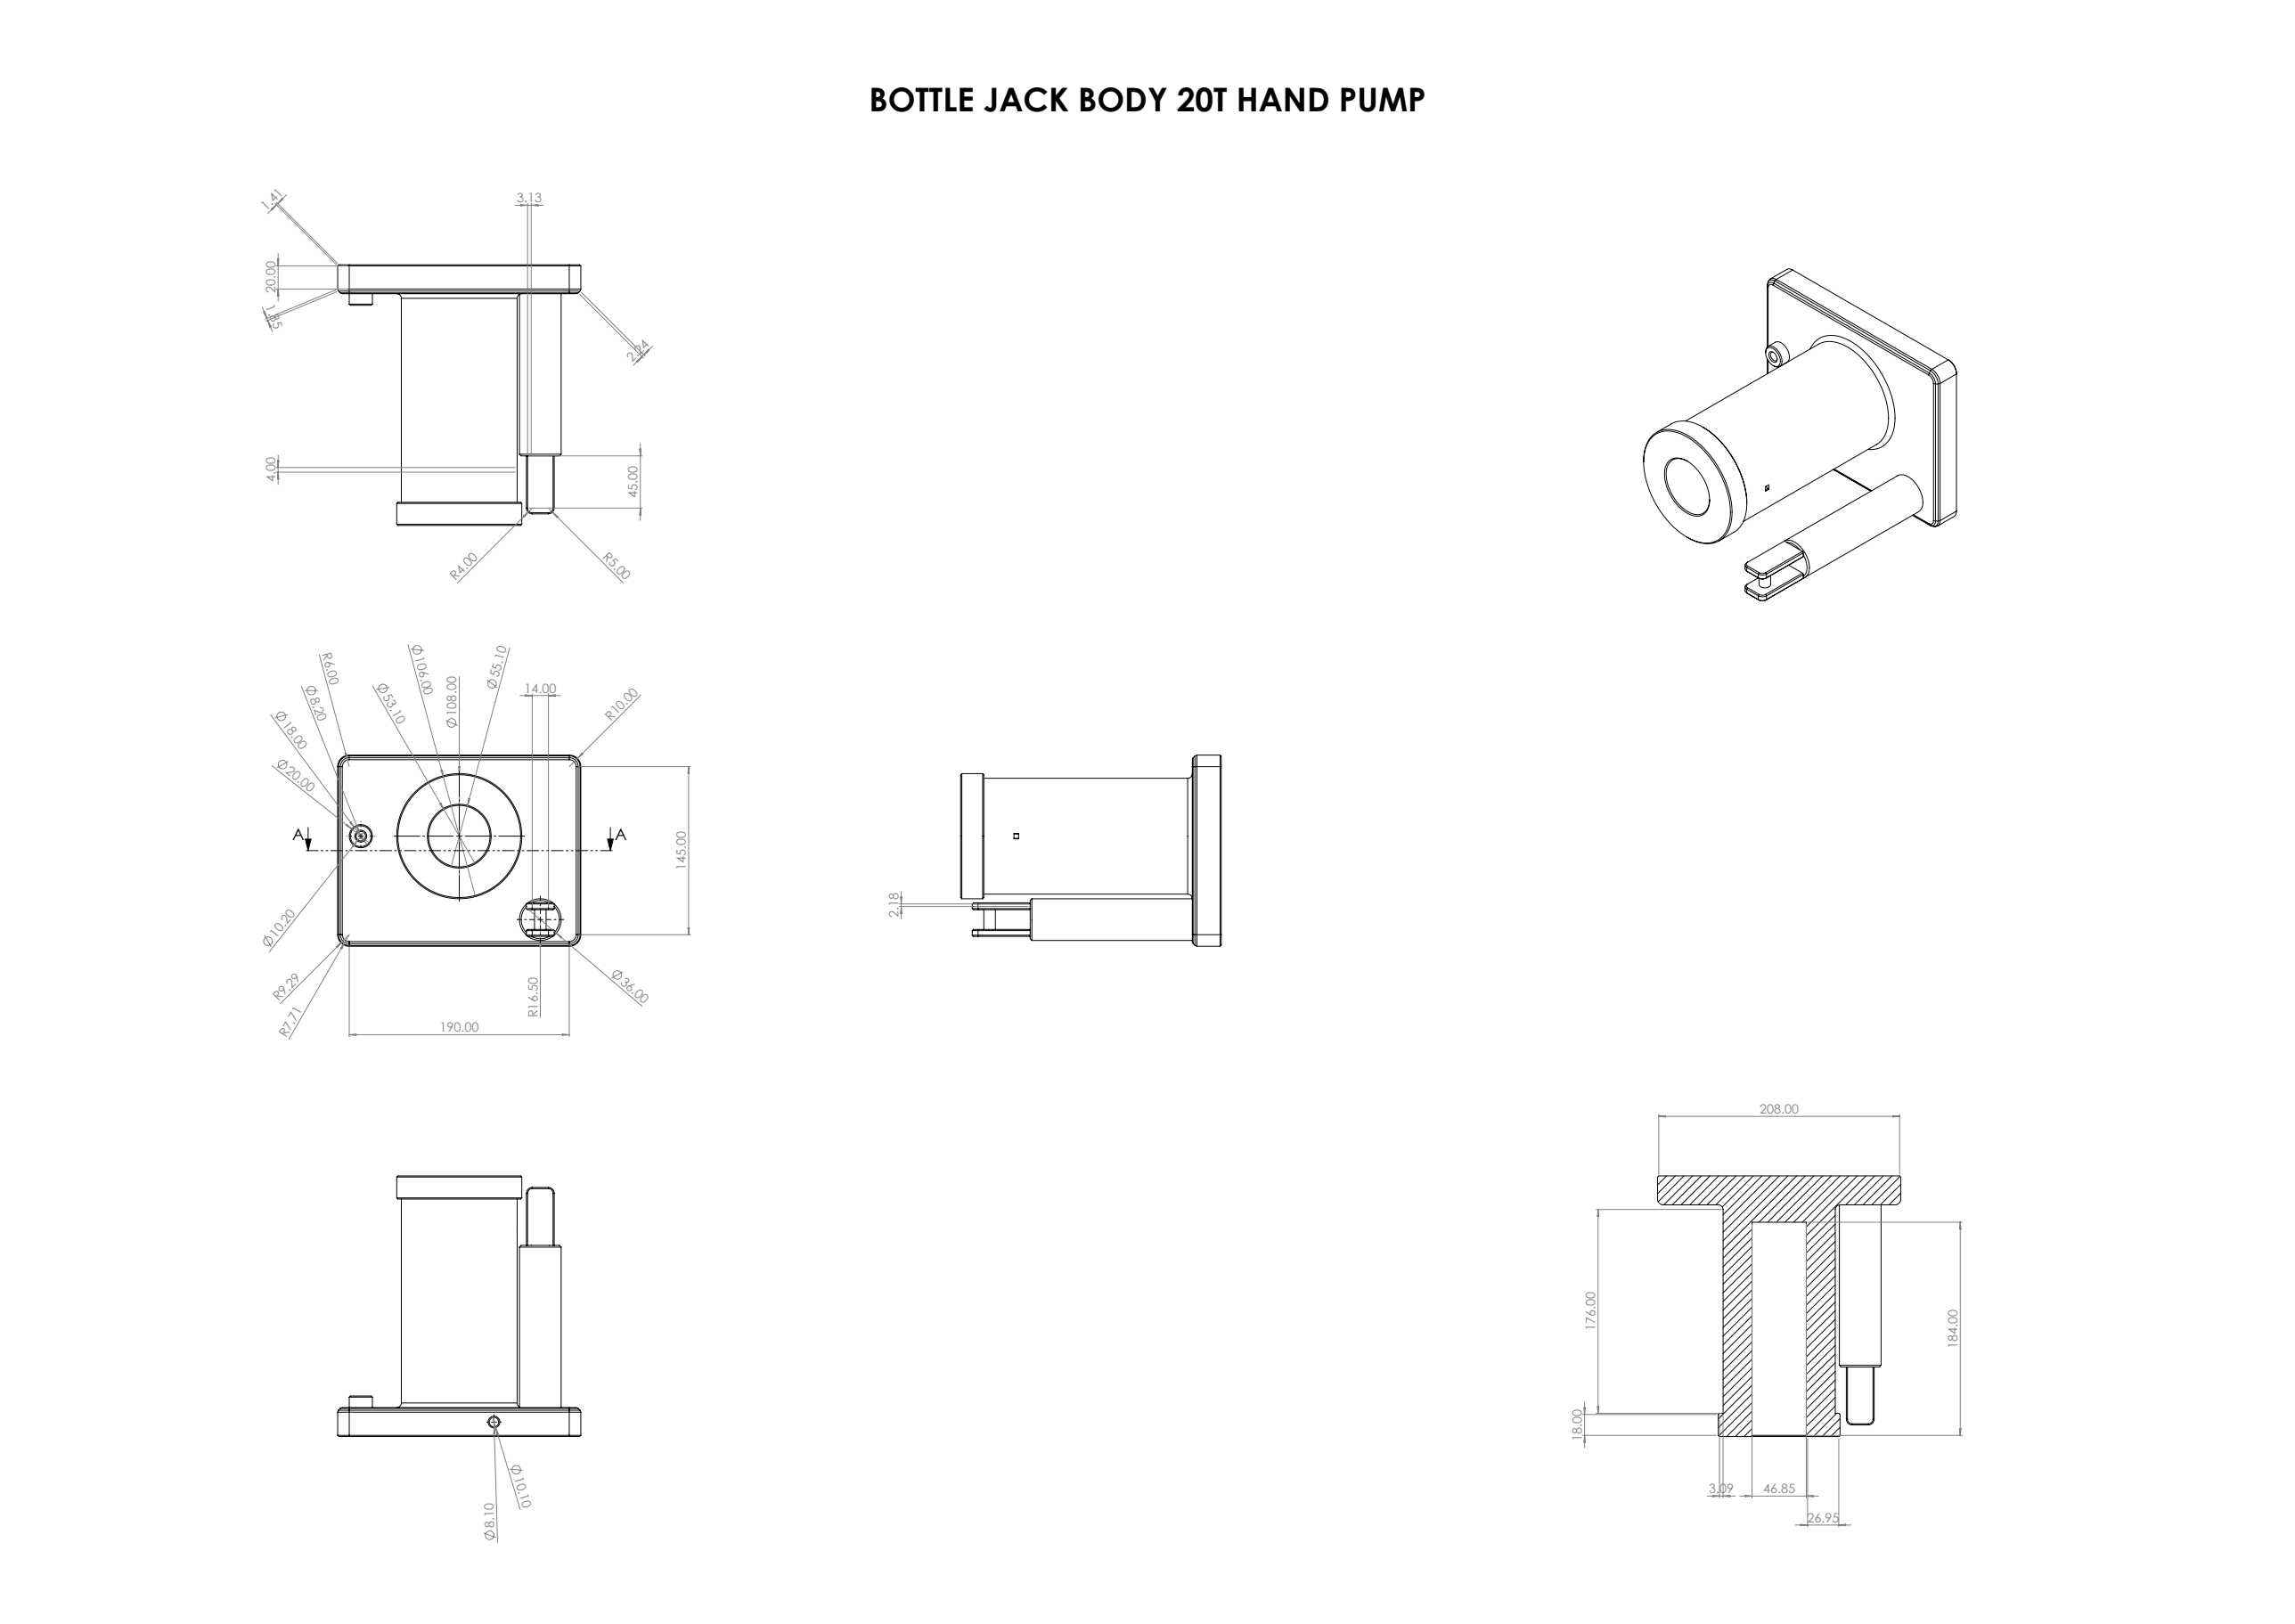
ISO-10303-21;
HEADER;
/* Generated by software containing ST-Developer
 * from STEP Tools, Inc. (www.steptools.com) 
 */

FILE_DESCRIPTION(
/* description */ (''),
/* implementation_level */ '2;1');

FILE_NAME(
/* name */ '09_Bottle_Jack_Body_20T_Hand_Pump.step',
/* time_stamp */ '2026-10-20T10:03:03-07:00',
/* author */ (''),
/* organization */ (''),
/* preprocessor_version */ 'ST-DEVELOPER v20.2',
/* originating_system */ 'Autodesk Translation Framework v15.15.0.0',
/* authorisation */ '');

FILE_SCHEMA (('AUTOMOTIVE_DESIGN { 1 0 10303 214 3 1 1 }'));
ENDSEC;

DATA;
#10=MECHANICAL_DESIGN_GEOMETRIC_PRESENTATION_REPRESENTATION('',(#528),#71492);
#376=TOROIDAL_SURFACE('',#29501,5.4,0.4);
#386=SHAPE_REPRESENTATION_RELATIONSHIP('SRR','None',#71607,#405);
#405=ADVANCED_BREP_SHAPE_REPRESENTATION('',(#424),#71477);
#424=MANIFOLD_SOLID_BREP('Jack body',#28463);
#528=STYLED_ITEM('',(#71866),#424);
#1575=CYLINDRICAL_SURFACE('',#29374,0.2);
#1576=CYLINDRICAL_SURFACE('',#29392,1.);
#1577=CYLINDRICAL_SURFACE('',#29395,1.);
#1578=CYLINDRICAL_SURFACE('',#29445,0.5);
#1579=CYLINDRICAL_SURFACE('',#29447,0.5);
#1580=CYLINDRICAL_SURFACE('',#29456,1.);
#1581=CYLINDRICAL_SURFACE('',#29459,0.41);
#1582=CYLINDRICAL_SURFACE('',#29463,0.405000000000001);
#1583=CYLINDRICAL_SURFACE('',#29467,0.5);
#1584=CYLINDRICAL_SURFACE('',#29468,0.5);
#1585=CYLINDRICAL_SURFACE('',#29470,0.5);
#1586=CYLINDRICAL_SURFACE('',#29488,1.8);
#1587=CYLINDRICAL_SURFACE('',#29492,2.655);
#1588=CYLINDRICAL_SURFACE('',#29505,5.);
#1589=CYLINDRICAL_SURFACE('',#29511,5.4);
#1590=CYLINDRICAL_SURFACE('',#29528,1.);
#1591=CYLINDRICAL_SURFACE('',#29533,1.);
#1918=FACE_BOUND('',#5174,.T.);
#1919=FACE_BOUND('',#5175,.T.);
#1920=FACE_BOUND('',#5176,.T.);
#1921=FACE_BOUND('',#5192,.T.);
#1922=FACE_BOUND('',#5208,.T.);
#1923=FACE_BOUND('',#5215,.T.);
#1924=FACE_BOUND('',#5229,.T.);
#1925=FACE_BOUND('',#5254,.T.);
#1926=FACE_BOUND('',#5260,.T.);
#1927=FACE_BOUND('',#5262,.T.);
#2238=CIRCLE('',#29348,0.770710678118652);
#2239=CIRCLE('',#29349,0.599999999999999);
#2240=CIRCLE('',#29352,0.770710678118652);
#2241=CIRCLE('',#29353,0.599999999999999);
#2242=CIRCLE('',#29356,0.770710678118652);
#2243=CIRCLE('',#29357,0.599999999999999);
#2244=CIRCLE('',#29360,0.770710678118652);
#2245=CIRCLE('',#29361,0.599999999999999);
#2246=CIRCLE('',#29365,0.929289321881342);
#2247=CIRCLE('',#29368,0.929289321881342);
#2248=CIRCLE('',#29370,5.4);
#2249=CIRCLE('',#29371,1.8);
#2250=CIRCLE('',#29372,1.);
#2251=CIRCLE('',#29375,0.2);
#2252=CIRCLE('',#29376,0.2);
#2253=CIRCLE('',#29380,1.);
#2254=CIRCLE('',#29383,0.929289321881336);
#2255=CIRCLE('',#29384,1.);
#2256=CIRCLE('',#29387,0.929289321881336);
#2257=CIRCLE('',#29388,1.);
#2258=CIRCLE('',#29391,1.);
#2259=CIRCLE('',#29393,1.);
#2260=CIRCLE('',#29396,1.);
#2261=CIRCLE('',#29398,0.504999999999995);
#2262=CIRCLE('',#29403,0.5);
#2263=CIRCLE('',#29404,0.400000000000011);
#2264=CIRCLE('',#29407,0.5);
#2265=CIRCLE('',#29408,0.400000000000012);
#2266=CIRCLE('',#29411,1.65);
#2267=CIRCLE('',#29415,0.5);
#2268=CIRCLE('',#29416,0.400000000000012);
#2269=CIRCLE('',#29419,0.5);
#2270=CIRCLE('',#29420,0.400000000000011);
#2271=CIRCLE('',#29423,0.5);
#2272=CIRCLE('',#29426,0.5);
#2273=CIRCLE('',#29427,0.400000000000011);
#2274=CIRCLE('',#29430,0.5);
#2275=CIRCLE('',#29431,0.400000000000012);
#2276=CIRCLE('',#29434,0.5);
#2277=CIRCLE('',#29437,0.5);
#2278=CIRCLE('',#29438,0.400000000000012);
#2279=CIRCLE('',#29441,0.5);
#2280=CIRCLE('',#29442,0.400000000000011);
#2281=CIRCLE('',#29450,1.65);
#2282=CIRCLE('',#29452,0.9);
#2283=CIRCLE('',#29453,1.);
#2284=CIRCLE('',#29455,0.51);
#2285=CIRCLE('',#29458,0.41);
#2286=CIRCLE('',#29460,0.41);
#2287=CIRCLE('',#29462,0.405000000000001);
#2288=CIRCLE('',#29464,0.405000000000001);
#2289=CIRCLE('',#29472,1.65);
#2290=CIRCLE('',#29476,1.65);
#2291=CIRCLE('',#29478,1.65);
#2292=CIRCLE('',#29481,1.65);
#2293=CIRCLE('',#29483,1.65);
#2294=CIRCLE('',#29484,1.65);
#2295=CIRCLE('',#29485,1.65);
#2296=CIRCLE('',#29487,1.8);
#2297=CIRCLE('',#29490,2.755);
#2298=CIRCLE('',#29491,2.655);
#2299=CIRCLE('',#29493,2.655);
#2300=CIRCLE('',#29495,5.3);
#2301=CIRCLE('',#29497,5.);
#2302=CIRCLE('',#29499,5.);
#2303=CIRCLE('',#29502,5.);
#2304=CIRCLE('',#29503,0.4);
#2305=CIRCLE('',#29504,5.);
#2306=CIRCLE('',#29506,5.);
#2307=CIRCLE('',#29508,5.3);
#2308=CIRCLE('',#29510,5.4);
#2309=CIRCLE('',#29512,5.4);
#2310=CIRCLE('',#29516,0.9);
#2311=CIRCLE('',#29519,1.);
#2312=CIRCLE('',#29520,0.9);
#2313=CIRCLE('',#29523,1.);
#2314=CIRCLE('',#29524,0.9);
#2315=CIRCLE('',#29527,0.9);
#2819=CONICAL_SURFACE('',#29347,0.685355339059325,1.17809724509615);
#2820=CONICAL_SURFACE('',#29351,0.685355339059325,1.17809724509615);
#2821=CONICAL_SURFACE('',#29355,0.685355339059325,1.17809724509615);
#2822=CONICAL_SURFACE('',#29359,0.685355339059325,1.17809724509615);
#2823=CONICAL_SURFACE('',#29364,0.85,0.785398163397452);
#2824=CONICAL_SURFACE('',#29367,0.85,0.785398163397452);
#2825=CONICAL_SURFACE('',#29379,0.964644660940671,0.392699081698743);
#2826=CONICAL_SURFACE('',#29382,0.964644660940668,0.392699081698775);
#2827=CONICAL_SURFACE('',#29386,0.964644660940668,0.392699081698775);
#2828=CONICAL_SURFACE('',#29390,0.964644660940671,0.392699081698743);
#2829=CONICAL_SURFACE('',#29399,0.85,0.785398163397452);
#2830=CONICAL_SURFACE('',#29402,0.450000000000006,0.785398163397392);
#2831=CONICAL_SURFACE('',#29406,0.450000000000006,0.785398163397389);
#2832=CONICAL_SURFACE('',#29414,0.450000000000006,0.785398163397389);
#2833=CONICAL_SURFACE('',#29418,0.450000000000006,0.785398163397392);
#2834=CONICAL_SURFACE('',#29425,0.450000000000006,0.785398163397392);
#2835=CONICAL_SURFACE('',#29429,0.450000000000006,0.785398163397389);
#2836=CONICAL_SURFACE('',#29436,0.450000000000006,0.785398163397389);
#2837=CONICAL_SURFACE('',#29440,0.450000000000006,0.785398163397392);
#2838=CONICAL_SURFACE('',#29451,0.95,0.785398163397475);
#2839=CONICAL_SURFACE('',#29457,0.46,0.785398163397475);
#2840=CONICAL_SURFACE('',#29461,0.454999999999998,0.785398163397422);
#2841=CONICAL_SURFACE('',#29465,0.405000000000001,1.02974425867666);
#2842=CONICAL_SURFACE('',#29466,0.205,1.02974425867666);
#2843=CONICAL_SURFACE('',#29486,1.725,0.785398163397431);
#2844=CONICAL_SURFACE('',#29489,2.705,0.785398163397477);
#2845=CONICAL_SURFACE('',#29509,5.35,0.785398163397479);
#2846=CONICAL_SURFACE('',#29513,5.35,0.785398163397479);
#2847=CONICAL_SURFACE('',#29515,0.95,0.785398163397475);
#2848=CONICAL_SURFACE('',#29518,0.95,0.785398163397475);
#2849=CONICAL_SURFACE('',#29522,0.95,0.785398163397475);
#2850=CONICAL_SURFACE('',#29526,0.95,0.785398163397475);
#2851=CONICAL_SURFACE('',#29531,0.85,0.785398163397452);
#3537=FACE_OUTER_BOUND('',#5161,.T.);
#3538=FACE_OUTER_BOUND('',#5162,.T.);
#3539=FACE_OUTER_BOUND('',#5163,.T.);
#3540=FACE_OUTER_BOUND('',#5164,.T.);
#3541=FACE_OUTER_BOUND('',#5165,.T.);
#3542=FACE_OUTER_BOUND('',#5166,.T.);
#3543=FACE_OUTER_BOUND('',#5167,.T.);
#3544=FACE_OUTER_BOUND('',#5168,.T.);
#3545=FACE_OUTER_BOUND('',#5169,.T.);
#3546=FACE_OUTER_BOUND('',#5170,.T.);
#3547=FACE_OUTER_BOUND('',#5171,.T.);
#3548=FACE_OUTER_BOUND('',#5172,.T.);
#3549=FACE_OUTER_BOUND('',#5173,.T.);
#3550=FACE_OUTER_BOUND('',#5177,.T.);
#3551=FACE_OUTER_BOUND('',#5178,.T.);
#3552=FACE_OUTER_BOUND('',#5179,.T.);
#3553=FACE_OUTER_BOUND('',#5180,.T.);
#3554=FACE_OUTER_BOUND('',#5181,.T.);
#3555=FACE_OUTER_BOUND('',#5182,.T.);
#3556=FACE_OUTER_BOUND('',#5183,.T.);
#3557=FACE_OUTER_BOUND('',#5184,.T.);
#3558=FACE_OUTER_BOUND('',#5185,.T.);
#3559=FACE_OUTER_BOUND('',#5186,.T.);
#3560=FACE_OUTER_BOUND('',#5187,.T.);
#3561=FACE_OUTER_BOUND('',#5188,.T.);
#3562=FACE_OUTER_BOUND('',#5189,.T.);
#3563=FACE_OUTER_BOUND('',#5190,.T.);
#3564=FACE_OUTER_BOUND('',#5191,.T.);
#3565=FACE_OUTER_BOUND('',#5193,.T.);
#3566=FACE_OUTER_BOUND('',#5194,.T.);
#3567=FACE_OUTER_BOUND('',#5195,.T.);
#3568=FACE_OUTER_BOUND('',#5196,.T.);
#3569=FACE_OUTER_BOUND('',#5197,.T.);
#3570=FACE_OUTER_BOUND('',#5198,.T.);
#3571=FACE_OUTER_BOUND('',#5199,.T.);
#3572=FACE_OUTER_BOUND('',#5200,.T.);
#3573=FACE_OUTER_BOUND('',#5201,.T.);
#3574=FACE_OUTER_BOUND('',#5202,.T.);
#3575=FACE_OUTER_BOUND('',#5203,.T.);
#3576=FACE_OUTER_BOUND('',#5204,.T.);
#3577=FACE_OUTER_BOUND('',#5205,.T.);
#3578=FACE_OUTER_BOUND('',#5206,.T.);
#3579=FACE_OUTER_BOUND('',#5207,.T.);
#3580=FACE_OUTER_BOUND('',#5209,.T.);
#3581=FACE_OUTER_BOUND('',#5210,.T.);
#3582=FACE_OUTER_BOUND('',#5211,.T.);
#3583=FACE_OUTER_BOUND('',#5212,.T.);
#3584=FACE_OUTER_BOUND('',#5213,.T.);
#3585=FACE_OUTER_BOUND('',#5214,.T.);
#3586=FACE_OUTER_BOUND('',#5216,.T.);
#3587=FACE_OUTER_BOUND('',#5217,.T.);
#3588=FACE_OUTER_BOUND('',#5218,.T.);
#3589=FACE_OUTER_BOUND('',#5219,.T.);
#3590=FACE_OUTER_BOUND('',#5220,.T.);
#3591=FACE_OUTER_BOUND('',#5221,.T.);
#3592=FACE_OUTER_BOUND('',#5222,.T.);
#3593=FACE_OUTER_BOUND('',#5223,.T.);
#3594=FACE_OUTER_BOUND('',#5224,.T.);
#3595=FACE_OUTER_BOUND('',#5225,.T.);
#3596=FACE_OUTER_BOUND('',#5226,.T.);
#3597=FACE_OUTER_BOUND('',#5227,.T.);
#3598=FACE_OUTER_BOUND('',#5228,.T.);
#3599=FACE_OUTER_BOUND('',#5230,.T.);
#3600=FACE_OUTER_BOUND('',#5231,.T.);
#3601=FACE_OUTER_BOUND('',#5232,.T.);
#3602=FACE_OUTER_BOUND('',#5233,.T.);
#3603=FACE_OUTER_BOUND('',#5234,.T.);
#3604=FACE_OUTER_BOUND('',#5235,.T.);
#3605=FACE_OUTER_BOUND('',#5236,.T.);
#3606=FACE_OUTER_BOUND('',#5237,.T.);
#3607=FACE_OUTER_BOUND('',#5238,.T.);
#3608=FACE_OUTER_BOUND('',#5239,.T.);
#3609=FACE_OUTER_BOUND('',#5240,.T.);
#3610=FACE_OUTER_BOUND('',#5241,.T.);
#3611=FACE_OUTER_BOUND('',#5242,.T.);
#3612=FACE_OUTER_BOUND('',#5243,.T.);
#3613=FACE_OUTER_BOUND('',#5244,.T.);
#3614=FACE_OUTER_BOUND('',#5245,.T.);
#3615=FACE_OUTER_BOUND('',#5246,.T.);
#3616=FACE_OUTER_BOUND('',#5247,.T.);
#3617=FACE_OUTER_BOUND('',#5248,.T.);
#3618=FACE_OUTER_BOUND('',#5249,.T.);
#3619=FACE_OUTER_BOUND('',#5250,.T.);
#3620=FACE_OUTER_BOUND('',#5251,.T.);
#3621=FACE_OUTER_BOUND('',#5252,.T.);
#3622=FACE_OUTER_BOUND('',#5253,.T.);
#3623=FACE_OUTER_BOUND('',#5255,.T.);
#3624=FACE_OUTER_BOUND('',#5256,.T.);
#3625=FACE_OUTER_BOUND('',#5257,.T.);
#3626=FACE_OUTER_BOUND('',#5258,.T.);
#3627=FACE_OUTER_BOUND('',#5259,.T.);
#3628=FACE_OUTER_BOUND('',#5261,.T.);
#3629=FACE_OUTER_BOUND('',#5263,.T.);
#3630=FACE_OUTER_BOUND('',#5264,.T.);
#3631=FACE_OUTER_BOUND('',#5265,.T.);
#3632=FACE_OUTER_BOUND('',#5266,.T.);
#3633=FACE_OUTER_BOUND('',#5267,.T.);
#3634=FACE_OUTER_BOUND('',#5268,.T.);
#3635=FACE_OUTER_BOUND('',#5269,.T.);
#3636=FACE_OUTER_BOUND('',#5270,.T.);
#3637=FACE_OUTER_BOUND('',#5271,.T.);
#3638=FACE_OUTER_BOUND('',#5272,.T.);
#3639=FACE_OUTER_BOUND('',#5273,.T.);
#3640=FACE_OUTER_BOUND('',#5274,.T.);
#3641=FACE_OUTER_BOUND('',#5275,.T.);
#3642=FACE_OUTER_BOUND('',#5276,.T.);
#3643=FACE_OUTER_BOUND('',#5277,.T.);
#3644=FACE_OUTER_BOUND('',#5278,.T.);
#3645=FACE_OUTER_BOUND('',#5279,.T.);
#3646=FACE_OUTER_BOUND('',#5280,.T.);
#5161=EDGE_LOOP('',(#20973,#20974,#20975,#20976));
#5162=EDGE_LOOP('',(#20977,#20978,#20979,#20980));
#5163=EDGE_LOOP('',(#20981,#20982,#20983,#20984));
#5164=EDGE_LOOP('',(#20985,#20986,#20987,#20988));
#5165=EDGE_LOOP('',(#20989,#20990,#20991,#20992));
#5166=EDGE_LOOP('',(#20993,#20994,#20995,#20996));
#5167=EDGE_LOOP('',(#20997,#20998,#20999,#21000));
#5168=EDGE_LOOP('',(#21001,#21002,#21003,#21004));
#5169=EDGE_LOOP('',(#21005,#21006,#21007,#21008));
#5170=EDGE_LOOP('',(#21009,#21010,#21011,#21012));
#5171=EDGE_LOOP('',(#21013,#21014,#21015,#21016));
#5172=EDGE_LOOP('',(#21017,#21018,#21019,#21020));
#5173=EDGE_LOOP('',(#21021,#21022,#21023,#21024,#21025,#21026,#21027,#21028));
#5174=EDGE_LOOP('',(#21029));
#5175=EDGE_LOOP('',(#21030));
#5176=EDGE_LOOP('',(#21031));
#5177=EDGE_LOOP('',(#21032,#21033,#21034,#21035));
#5178=EDGE_LOOP('',(#21036,#21037,#21038,#21039));
#5179=EDGE_LOOP('',(#21040,#21041,#21042,#21043));
#5180=EDGE_LOOP('',(#21044,#21045,#21046,#21047));
#5181=EDGE_LOOP('',(#21048,#21049,#21050,#21051));
#5182=EDGE_LOOP('',(#21052,#21053,#21054,#21055));
#5183=EDGE_LOOP('',(#21056,#21057,#21058,#21059));
#5184=EDGE_LOOP('',(#21060,#21061,#21062,#21063));
#5185=EDGE_LOOP('',(#21064,#21065,#21066,#21067));
#5186=EDGE_LOOP('',(#21068,#21069,#21070,#21071));
#5187=EDGE_LOOP('',(#21072,#21073,#21074,#21075));
#5188=EDGE_LOOP('',(#21076,#21077,#21078,#21079));
#5189=EDGE_LOOP('',(#21080,#21081,#21082,#21083));
#5190=EDGE_LOOP('',(#21084,#21085,#21086,#21087));
#5191=EDGE_LOOP('',(#21088,#21089,#21090,#21091));
#5192=EDGE_LOOP('',(#21092));
#5193=EDGE_LOOP('',(#21093,#21094,#21095,#21096));
#5194=EDGE_LOOP('',(#21097,#21098,#21099,#21100));
#5195=EDGE_LOOP('',(#21101,#21102,#21103,#21104));
#5196=EDGE_LOOP('',(#21105,#21106,#21107,#21108));
#5197=EDGE_LOOP('',(#21109,#21110,#21111,#21112));
#5198=EDGE_LOOP('',(#21113,#21114,#21115,#21116));
#5199=EDGE_LOOP('',(#21117,#21118,#21119,#21120));
#5200=EDGE_LOOP('',(#21121,#21122,#21123,#21124));
#5201=EDGE_LOOP('',(#21125,#21126,#21127,#21128,#21129,#21130,#21131,#21132));
#5202=EDGE_LOOP('',(#21133,#21134,#21135,#21136));
#5203=EDGE_LOOP('',(#21137,#21138,#21139,#21140));
#5204=EDGE_LOOP('',(#21141,#21142,#21143,#21144));
#5205=EDGE_LOOP('',(#21145,#21146,#21147,#21148));
#5206=EDGE_LOOP('',(#21149,#21150,#21151,#21152));
#5207=EDGE_LOOP('',(#21153,#21154,#21155,#21156,#21157,#21158));
#5208=EDGE_LOOP('',(#21159));
#5209=EDGE_LOOP('',(#21160,#21161,#21162,#21163));
#5210=EDGE_LOOP('',(#21164,#21165,#21166,#21167));
#5211=EDGE_LOOP('',(#21168,#21169,#21170,#21171));
#5212=EDGE_LOOP('',(#21172,#21173,#21174,#21175));
#5213=EDGE_LOOP('',(#21176,#21177,#21178,#21179));
#5214=EDGE_LOOP('',(#21180,#21181,#21182,#21183,#21184,#21185));
#5215=EDGE_LOOP('',(#21186));
#5216=EDGE_LOOP('',(#21187,#21188,#21189,#21190));
#5217=EDGE_LOOP('',(#21191,#21192,#21193,#21194));
#5218=EDGE_LOOP('',(#21195,#21196,#21197,#21198));
#5219=EDGE_LOOP('',(#21199,#21200,#21201,#21202));
#5220=EDGE_LOOP('',(#21203,#21204,#21205,#21206));
#5221=EDGE_LOOP('',(#21207,#21208,#21209,#21210,#21211));
#5222=EDGE_LOOP('',(#21212,#21213,#21214,#21215));
#5223=EDGE_LOOP('',(#21216,#21217,#21218,#21219));
#5224=EDGE_LOOP('',(#21220,#21221,#21222,#21223));
#5225=EDGE_LOOP('',(#21224,#21225,#21226,#21227,#21228));
#5226=EDGE_LOOP('',(#21229,#21230,#21231,#21232));
#5227=EDGE_LOOP('',(#21233,#21234,#21235,#21236));
#5228=EDGE_LOOP('',(#21237));
#5229=EDGE_LOOP('',(#21238));
#5230=EDGE_LOOP('',(#21239,#21240,#21241,#21242));
#5231=EDGE_LOOP('',(#21243,#21244,#21245,#21246));
#5232=EDGE_LOOP('',(#21247,#21248,#21249,#21250));
#5233=EDGE_LOOP('',(#21251,#21252,#21253,#21254));
#5234=EDGE_LOOP('',(#21255,#21256,#21257,#21258));
#5235=EDGE_LOOP('',(#21259,#21260,#21261));
#5236=EDGE_LOOP('',(#21262,#21263,#21264));
#5237=EDGE_LOOP('',(#21265,#21266,#21267,#21268));
#5238=EDGE_LOOP('',(#21269,#21270,#21271,#21272));
#5239=EDGE_LOOP('',(#21273,#21274,#21275,#21276));
#5240=EDGE_LOOP('',(#21277,#21278,#21279,#21280));
#5241=EDGE_LOOP('',(#21281,#21282,#21283,#21284));
#5242=EDGE_LOOP('',(#21285,#21286,#21287,#21288,#21289));
#5243=EDGE_LOOP('',(#21290,#21291,#21292,#21293,#21294));
#5244=EDGE_LOOP('',(#21295,#21296));
#5245=EDGE_LOOP('',(#21297,#21298,#21299,#21300));
#5246=EDGE_LOOP('',(#21301,#21302,#21303,#21304,#21305,#21306,#21307,#21308));
#5247=EDGE_LOOP('',(#21309,#21310));
#5248=EDGE_LOOP('',(#21311,#21312,#21313,#21314,#21315,#21316,#21317,#21318,
#21319,#21320,#21321,#21322,#21323));
#5249=EDGE_LOOP('',(#21324,#21325,#21326,#21327,#21328,#21329,#21330,#21331,
#21332,#21333,#21334,#21335));
#5250=EDGE_LOOP('',(#21336,#21337,#21338,#21339));
#5251=EDGE_LOOP('',(#21340,#21341,#21342,#21343));
#5252=EDGE_LOOP('',(#21344,#21345,#21346,#21347));
#5253=EDGE_LOOP('',(#21348));
#5254=EDGE_LOOP('',(#21349));
#5255=EDGE_LOOP('',(#21350,#21351,#21352,#21353));
#5256=EDGE_LOOP('',(#21354,#21355,#21356,#21357));
#5257=EDGE_LOOP('',(#21358));
#5258=EDGE_LOOP('',(#21359,#21360,#21361,#21362,#21363));
#5259=EDGE_LOOP('',(#21364,#21365,#21366,#21367,#21368));
#5260=EDGE_LOOP('',(#21369,#21370,#21371,#21372));
#5261=EDGE_LOOP('',(#21373));
#5262=EDGE_LOOP('',(#21374));
#5263=EDGE_LOOP('',(#21375,#21376,#21377,#21378));
#5264=EDGE_LOOP('',(#21379,#21380,#21381,#21382));
#5265=EDGE_LOOP('',(#21383,#21384,#21385,#21386));
#5266=EDGE_LOOP('',(#21387,#21388,#21389,#21390));
#5267=EDGE_LOOP('',(#21391,#21392,#21393,#21394));
#5268=EDGE_LOOP('',(#21395,#21396,#21397,#21398));
#5269=EDGE_LOOP('',(#21399,#21400,#21401,#21402));
#5270=EDGE_LOOP('',(#21403,#21404,#21405,#21406));
#5271=EDGE_LOOP('',(#21407,#21408,#21409,#21410));
#5272=EDGE_LOOP('',(#21411,#21412,#21413,#21414));
#5273=EDGE_LOOP('',(#21415,#21416,#21417,#21418));
#5274=EDGE_LOOP('',(#21419,#21420,#21421,#21422));
#5275=EDGE_LOOP('',(#21423,#21424,#21425,#21426,#21427,#21428,#21429,#21430));
#5276=EDGE_LOOP('',(#21431,#21432,#21433,#21434));
#5277=EDGE_LOOP('',(#21435,#21436,#21437,#21438));
#5278=EDGE_LOOP('',(#21439,#21440,#21441,#21442));
#5279=EDGE_LOOP('',(#21443,#21444,#21445,#21446));
#5280=EDGE_LOOP('',(#21447,#21448,#21449,#21450));
#7402=LINE('',#43533,#9890);
#7403=LINE('',#43537,#9891);
#7404=LINE('',#43542,#9892);
#7405=LINE('',#43543,#9893);
#7406=LINE('',#43544,#9894);
#7407=LINE('',#43548,#9895);
#7408=LINE('',#43554,#9896);
#7409=LINE('',#43555,#9897);
#7410=LINE('',#43556,#9898);
#7411=LINE('',#43560,#9899);
#7412=LINE('',#43566,#9900);
#7413=LINE('',#43567,#9901);
#7414=LINE('',#43568,#9902);
#7415=LINE('',#43572,#9903);
#7416=LINE('',#43576,#9904);
#7417=LINE('',#43577,#9905);
#7418=LINE('',#43580,#9906);
#7419=LINE('',#43582,#9907);
#7420=LINE('',#43583,#9908);
#7421=LINE('',#43586,#9909);
#7422=LINE('',#43590,#9910);
#7423=LINE('',#43591,#9911);
#7424=LINE('',#43594,#9912);
#7425=LINE('',#43606,#9913);
#7426=LINE('',#43608,#9914);
#7427=LINE('',#43610,#9915);
#7428=LINE('',#43611,#9916);
#7429=LINE('',#43616,#9917);
#7430=LINE('',#43620,#9918);
#7431=LINE('',#43622,#9919);
#7432=LINE('',#43623,#9920);
#7433=LINE('',#43626,#9921);
#7434=LINE('',#43628,#9922);
#7435=LINE('',#43629,#9923);
#7436=LINE('',#43632,#9924);
#7437=LINE('',#43636,#9925);
#7438=LINE('',#43637,#9926);
#7439=LINE('',#43641,#9927);
#7440=LINE('',#43647,#9928);
#7441=LINE('',#43648,#9929);
#7442=LINE('',#43649,#9930);
#7443=LINE('',#43653,#9931);
#7444=LINE('',#43658,#9932);
#7445=LINE('',#43659,#9933);
#7446=LINE('',#43660,#9934);
#7447=LINE('',#43665,#9935);
#7448=LINE('',#43668,#9936);
#7449=LINE('',#43671,#9937);
#7450=LINE('',#43672,#9938);
#7451=LINE('',#43675,#9939);
#7452=LINE('',#43679,#9940);
#7453=LINE('',#43680,#9941);
#7454=LINE('',#43684,#9942);
#7455=LINE('',#43685,#9943);
#7456=LINE('',#43690,#9944);
#7457=LINE('',#43692,#9945);
#7458=LINE('',#43694,#9946);
#7459=LINE('',#43695,#9947);
#7460=LINE('',#43699,#9948);
#7461=LINE('',#43705,#9949);
#7462=LINE('',#43706,#9950);
#7463=LINE('',#43707,#9951);
#7464=LINE('',#43711,#9952);
#7465=LINE('',#43717,#9953);
#7466=LINE('',#43718,#9954);
#7467=LINE('',#43719,#9955);
#7468=LINE('',#43722,#9956);
#7469=LINE('',#43725,#9957);
#7470=LINE('',#43728,#9958);
#7471=LINE('',#43729,#9959);
#7472=LINE('',#43733,#9960);
#7473=LINE('',#43735,#9961);
#7474=LINE('',#43737,#9962);
#7475=LINE('',#43738,#9963);
#7476=LINE('',#43742,#9964);
#7477=LINE('',#43748,#9965);
#7478=LINE('',#43749,#9966);
#7479=LINE('',#43750,#9967);
#7480=LINE('',#43754,#9968);
#7481=LINE('',#43760,#9969);
#7482=LINE('',#43761,#9970);
#7483=LINE('',#43762,#9971);
#7484=LINE('',#43764,#9972);
#7485=LINE('',#43770,#9973);
#7486=LINE('',#43772,#9974);
#7487=LINE('',#43774,#9975);
#7488=LINE('',#43775,#9976);
#7489=LINE('',#43779,#9977);
#7490=LINE('',#43785,#9978);
#7491=LINE('',#43786,#9979);
#7492=LINE('',#43787,#9980);
#7493=LINE('',#43791,#9981);
#7494=LINE('',#43797,#9982);
#7495=LINE('',#43798,#9983);
#7496=LINE('',#43799,#9984);
#7497=LINE('',#43801,#9985);
#7498=LINE('',#43807,#9986);
#7499=LINE('',#43809,#9987);
#7500=LINE('',#43811,#9988);
#7501=LINE('',#43812,#9989);
#7502=LINE('',#43816,#9990);
#7503=LINE('',#43822,#9991);
#7504=LINE('',#43823,#9992);
#7505=LINE('',#43824,#9993);
#7506=LINE('',#43828,#9994);
#7507=LINE('',#43834,#9995);
#7508=LINE('',#43835,#9996);
#7509=LINE('',#43836,#9997);
#7510=LINE('',#43839,#9998);
#7511=LINE('',#43840,#9999);
#7512=LINE('',#43841,#10000);
#7513=LINE('',#43843,#10001);
#7514=LINE('',#43845,#10002);
#7515=LINE('',#43847,#10003);
#7516=LINE('',#43850,#10004);
#7517=LINE('',#43851,#10005);
#7518=LINE('',#43854,#10006);
#7519=LINE('',#43860,#10007);
#7520=LINE('',#43866,#10008);
#7521=LINE('',#43869,#10009);
#7522=LINE('',#43874,#10010);
#7523=LINE('',#43877,#10011);
#7524=LINE('',#43881,#10012);
#7525=LINE('',#43885,#10013);
#7526=LINE('',#43888,#10014);
#7527=LINE('',#43890,#10015);
#7528=LINE('',#43892,#10016);
#7529=LINE('',#43893,#10017);
#7530=LINE('',#43895,#10018);
#7531=LINE('',#43897,#10019);
#7532=LINE('',#43900,#10020);
#7533=LINE('',#43903,#10021);
#7534=LINE('',#43905,#10022);
#7535=LINE('',#43911,#10023);
#7536=LINE('',#43913,#10024);
#7537=LINE('',#43923,#10025);
#7538=LINE('',#43926,#10026);
#7539=LINE('',#43931,#10027);
#7540=LINE('',#43936,#10028);
#7541=LINE('',#43954,#10029);
#7542=LINE('',#43961,#10030);
#7543=LINE('',#43965,#10031);
#7544=LINE('',#43967,#10032);
#7545=LINE('',#43970,#10033);
#7546=LINE('',#43972,#10034);
#7547=LINE('',#43973,#10035);
#7548=LINE('',#43976,#10036);
#7549=LINE('',#43981,#10037);
#7550=LINE('',#43982,#10038);
#7551=LINE('',#43983,#10039);
#7552=LINE('',#43987,#10040);
#7553=LINE('',#43993,#10041);
#7554=LINE('',#43994,#10042);
#7555=LINE('',#43995,#10043);
#7556=LINE('',#43998,#10044);
#7557=LINE('',#44003,#10045);
#7558=LINE('',#44004,#10046);
#7559=LINE('',#44008,#10047);
#7560=LINE('',#44011,#10048);
#7561=LINE('',#44014,#10049);
#7562=LINE('',#44016,#10050);
#9890=VECTOR('',#33275,1.);
#9891=VECTOR('',#33278,1.);
#9892=VECTOR('',#33283,1.);
#9893=VECTOR('',#33284,1.);
#9894=VECTOR('',#33285,1.);
#9895=VECTOR('',#33288,1.);
#9896=VECTOR('',#33295,1.);
#9897=VECTOR('',#33296,1.);
#9898=VECTOR('',#33297,1.);
#9899=VECTOR('',#33300,1.);
#9900=VECTOR('',#33307,1.);
#9901=VECTOR('',#33308,1.);
#9902=VECTOR('',#33309,1.);
#9903=VECTOR('',#33312,1.);
#9904=VECTOR('',#33319,1.);
#9905=VECTOR('',#33320,1.);
#9906=VECTOR('',#33323,1.);
#9907=VECTOR('',#33324,1.);
#9908=VECTOR('',#33325,1.);
#9909=VECTOR('',#33328,1.);
#9910=VECTOR('',#33333,1.);
#9911=VECTOR('',#33334,1.);
#9912=VECTOR('',#33337,1.);
#9913=VECTOR('',#33350,1.);
#9914=VECTOR('',#33351,1.);
#9915=VECTOR('',#33352,1.);
#9916=VECTOR('',#33353,1.);
#9917=VECTOR('',#33358,1.);
#9918=VECTOR('',#33363,1.);
#9919=VECTOR('',#33364,1.);
#9920=VECTOR('',#33365,1.);
#9921=VECTOR('',#33368,1.);
#9922=VECTOR('',#33369,1.);
#9923=VECTOR('',#33370,1.);
#9924=VECTOR('',#33373,1.);
#9925=VECTOR('',#33378,1.);
#9926=VECTOR('',#33379,1.);
#9927=VECTOR('',#33382,1.);
#9928=VECTOR('',#33389,1.);
#9929=VECTOR('',#33390,1.);
#9930=VECTOR('',#33391,1.);
#9931=VECTOR('',#33394,1.);
#9932=VECTOR('',#33401,1.);
#9933=VECTOR('',#33402,1.);
#9934=VECTOR('',#33403,1.);
#9935=VECTOR('',#33410,1.);
#9936=VECTOR('',#33413,1.);
#9937=VECTOR('',#33416,1.);
#9938=VECTOR('',#33417,1.);
#9939=VECTOR('',#33420,1.);
#9940=VECTOR('',#33425,1.);
#9941=VECTOR('',#33426,1.);
#9942=VECTOR('',#33431,1.);
#9943=VECTOR('',#33432,1.);
#9944=VECTOR('',#33437,1.);
#9945=VECTOR('',#33438,1.);
#9946=VECTOR('',#33439,1.);
#9947=VECTOR('',#33440,1.);
#9948=VECTOR('',#33443,1.);
#9949=VECTOR('',#33450,1.);
#9950=VECTOR('',#33451,1.);
#9951=VECTOR('',#33452,1.);
#9952=VECTOR('',#33455,1.);
#9953=VECTOR('',#33462,1.);
#9954=VECTOR('',#33463,1.);
#9955=VECTOR('',#33464,1.);
#9956=VECTOR('',#33467,1.);
#9957=VECTOR('',#33470,1.);
#9958=VECTOR('',#33473,1.);
#9959=VECTOR('',#33474,1.);
#9960=VECTOR('',#33477,1.);
#9961=VECTOR('',#33478,1.);
#9962=VECTOR('',#33479,1.);
#9963=VECTOR('',#33480,1.);
#9964=VECTOR('',#33483,1.);
#9965=VECTOR('',#33490,1.);
#9966=VECTOR('',#33491,1.);
#9967=VECTOR('',#33492,1.);
#9968=VECTOR('',#33495,1.);
#9969=VECTOR('',#33502,1.);
#9970=VECTOR('',#33503,1.);
#9971=VECTOR('',#33504,1.);
#9972=VECTOR('',#33507,1.);
#9973=VECTOR('',#33512,1.);
#9974=VECTOR('',#33513,1.);
#9975=VECTOR('',#33514,1.);
#9976=VECTOR('',#33515,1.);
#9977=VECTOR('',#33518,1.);
#9978=VECTOR('',#33525,1.);
#9979=VECTOR('',#33526,1.);
#9980=VECTOR('',#33527,1.);
#9981=VECTOR('',#33530,1.);
#9982=VECTOR('',#33537,1.);
#9983=VECTOR('',#33538,1.);
#9984=VECTOR('',#33539,1.);
#9985=VECTOR('',#33542,1.);
#9986=VECTOR('',#33547,1.);
#9987=VECTOR('',#33548,1.);
#9988=VECTOR('',#33549,1.);
#9989=VECTOR('',#33550,1.);
#9990=VECTOR('',#33553,1.);
#9991=VECTOR('',#33560,1.);
#9992=VECTOR('',#33561,1.);
#9993=VECTOR('',#33562,1.);
#9994=VECTOR('',#33565,1.);
#9995=VECTOR('',#33572,1.);
#9996=VECTOR('',#33573,1.);
#9997=VECTOR('',#33574,1.);
#9998=VECTOR('',#33577,1.);
#9999=VECTOR('',#33578,1.);
#10000=VECTOR('',#33579,1.);
#10001=VECTOR('',#33582,1.);
#10002=VECTOR('',#33585,1.);
#10003=VECTOR('',#33588,1.);
#10004=VECTOR('',#33591,1.);
#10005=VECTOR('',#33592,1.);
#10006=VECTOR('',#33595,1.);
#10007=VECTOR('',#33602,0.95);
#10008=VECTOR('',#33611,1.);
#10009=VECTOR('',#33614,0.46);
#10010=VECTOR('',#33621,0.41);
#10011=VECTOR('',#33624,0.454999999999998);
#10012=VECTOR('',#33629,0.405000000000001);
#10013=VECTOR('',#33634,0.405000000000001);
#10014=VECTOR('',#33637,0.205);
#10015=VECTOR('',#33640,0.5);
#10016=VECTOR('',#33643,1.);
#10017=VECTOR('',#33644,1.);
#10018=VECTOR('',#33647,1.);
#10019=VECTOR('',#33650,1.);
#10020=VECTOR('',#33653,1.);
#10021=VECTOR('',#33658,1.);
#10022=VECTOR('',#33661,1.);
#10023=VECTOR('',#33670,1.);
#10024=VECTOR('',#33673,1.);
#10025=VECTOR('',#33688,1.725);
#10026=VECTOR('',#33693,1.8);
#10027=VECTOR('',#33698,2.705);
#10028=VECTOR('',#33705,2.655);
#10029=VECTOR('',#33732,5.);
#10030=VECTOR('',#33741,5.35);
#10031=VECTOR('',#33746,5.4);
#10032=VECTOR('',#33749,5.35);
#10033=VECTOR('',#33752,1.);
#10034=VECTOR('',#33753,1.);
#10035=VECTOR('',#33754,1.);
#10036=VECTOR('',#33757,1.);
#10037=VECTOR('',#33762,1.);
#10038=VECTOR('',#33763,1.);
#10039=VECTOR('',#33764,1.);
#10040=VECTOR('',#33767,1.);
#10041=VECTOR('',#33774,1.);
#10042=VECTOR('',#33775,1.);
#10043=VECTOR('',#33776,1.);
#10044=VECTOR('',#33779,1.);
#10045=VECTOR('',#33786,1.);
#10046=VECTOR('',#33787,1.);
#10047=VECTOR('',#33794,1.);
#10048=VECTOR('',#33799,1.);
#10049=VECTOR('',#33804,1.);
#10050=VECTOR('',#33807,1.);
#12235=VERTEX_POINT('',#43531);
#12236=VERTEX_POINT('',#43532);
#12237=VERTEX_POINT('',#43534);
#12238=VERTEX_POINT('',#43536);
#12239=VERTEX_POINT('',#43540);
#12240=VERTEX_POINT('',#43541);
#12241=VERTEX_POINT('',#43546);
#12242=VERTEX_POINT('',#43547);
#12243=VERTEX_POINT('',#43552);
#12244=VERTEX_POINT('',#43553);
#12245=VERTEX_POINT('',#43558);
#12246=VERTEX_POINT('',#43559);
#12247=VERTEX_POINT('',#43564);
#12248=VERTEX_POINT('',#43565);
#12249=VERTEX_POINT('',#43570);
#12250=VERTEX_POINT('',#43571);
#12251=VERTEX_POINT('',#43579);
#12252=VERTEX_POINT('',#43581);
#12253=VERTEX_POINT('',#43585);
#12254=VERTEX_POINT('',#43589);
#12255=VERTEX_POINT('',#43593);
#12256=VERTEX_POINT('',#43597);
#12257=VERTEX_POINT('',#43599);
#12258=VERTEX_POINT('',#43601);
#12259=VERTEX_POINT('',#43604);
#12260=VERTEX_POINT('',#43605);
#12261=VERTEX_POINT('',#43607);
#12262=VERTEX_POINT('',#43609);
#12263=VERTEX_POINT('',#43613);
#12264=VERTEX_POINT('',#43615);
#12265=VERTEX_POINT('',#43619);
#12266=VERTEX_POINT('',#43621);
#12267=VERTEX_POINT('',#43625);
#12268=VERTEX_POINT('',#43627);
#12269=VERTEX_POINT('',#43631);
#12270=VERTEX_POINT('',#43635);
#12271=VERTEX_POINT('',#43639);
#12272=VERTEX_POINT('',#43640);
#12273=VERTEX_POINT('',#43645);
#12274=VERTEX_POINT('',#43646);
#12275=VERTEX_POINT('',#43651);
#12276=VERTEX_POINT('',#43652);
#12277=VERTEX_POINT('',#43657);
#12278=VERTEX_POINT('',#43664);
#12279=VERTEX_POINT('',#43666);
#12280=VERTEX_POINT('',#43670);
#12281=VERTEX_POINT('',#43674);
#12282=VERTEX_POINT('',#43678);
#12283=VERTEX_POINT('',#43681);
#12284=VERTEX_POINT('',#43688);
#12285=VERTEX_POINT('',#43689);
#12286=VERTEX_POINT('',#43691);
#12287=VERTEX_POINT('',#43693);
#12288=VERTEX_POINT('',#43697);
#12289=VERTEX_POINT('',#43698);
#12290=VERTEX_POINT('',#43703);
#12291=VERTEX_POINT('',#43704);
#12292=VERTEX_POINT('',#43709);
#12293=VERTEX_POINT('',#43710);
#12294=VERTEX_POINT('',#43715);
#12295=VERTEX_POINT('',#43716);
#12296=VERTEX_POINT('',#43721);
#12297=VERTEX_POINT('',#43723);
#12298=VERTEX_POINT('',#43727);
#12299=VERTEX_POINT('',#43731);
#12300=VERTEX_POINT('',#43732);
#12301=VERTEX_POINT('',#43734);
#12302=VERTEX_POINT('',#43736);
#12303=VERTEX_POINT('',#43740);
#12304=VERTEX_POINT('',#43741);
#12305=VERTEX_POINT('',#43746);
#12306=VERTEX_POINT('',#43747);
#12307=VERTEX_POINT('',#43752);
#12308=VERTEX_POINT('',#43753);
#12309=VERTEX_POINT('',#43758);
#12310=VERTEX_POINT('',#43759);
#12311=VERTEX_POINT('',#43765);
#12312=VERTEX_POINT('',#43768);
#12313=VERTEX_POINT('',#43769);
#12314=VERTEX_POINT('',#43771);
#12315=VERTEX_POINT('',#43773);
#12316=VERTEX_POINT('',#43777);
#12317=VERTEX_POINT('',#43778);
#12318=VERTEX_POINT('',#43783);
#12319=VERTEX_POINT('',#43784);
#12320=VERTEX_POINT('',#43789);
#12321=VERTEX_POINT('',#43790);
#12322=VERTEX_POINT('',#43795);
#12323=VERTEX_POINT('',#43796);
#12324=VERTEX_POINT('',#43802);
#12325=VERTEX_POINT('',#43805);
#12326=VERTEX_POINT('',#43806);
#12327=VERTEX_POINT('',#43808);
#12328=VERTEX_POINT('',#43810);
#12329=VERTEX_POINT('',#43814);
#12330=VERTEX_POINT('',#43815);
#12331=VERTEX_POINT('',#43820);
#12332=VERTEX_POINT('',#43821);
#12333=VERTEX_POINT('',#43826);
#12334=VERTEX_POINT('',#43827);
#12335=VERTEX_POINT('',#43832);
#12336=VERTEX_POINT('',#43833);
#12337=VERTEX_POINT('',#43838);
#12338=VERTEX_POINT('',#43849);
#12339=VERTEX_POINT('',#43853);
#12340=VERTEX_POINT('',#43857);
#12341=VERTEX_POINT('',#43859);
#12342=VERTEX_POINT('',#43863);
#12343=VERTEX_POINT('',#43868);
#12344=VERTEX_POINT('',#43872);
#12345=VERTEX_POINT('',#43876);
#12346=VERTEX_POINT('',#43880);
#12347=VERTEX_POINT('',#43884);
#12348=VERTEX_POINT('',#43887);
#12349=VERTEX_POINT('',#43899);
#12350=VERTEX_POINT('',#43909);
#12351=VERTEX_POINT('',#43917);
#12352=VERTEX_POINT('',#43922);
#12353=VERTEX_POINT('',#43928);
#12354=VERTEX_POINT('',#43930);
#12355=VERTEX_POINT('',#43934);
#12356=VERTEX_POINT('',#43938);
#12357=VERTEX_POINT('',#43946);
#12358=VERTEX_POINT('',#43947);
#12359=VERTEX_POINT('',#43952);
#12360=VERTEX_POINT('',#43956);
#12361=VERTEX_POINT('',#43959);
#12362=VERTEX_POINT('',#43963);
#12363=VERTEX_POINT('',#43969);
#12364=VERTEX_POINT('',#43971);
#12365=VERTEX_POINT('',#43975);
#12366=VERTEX_POINT('',#43979);
#12367=VERTEX_POINT('',#43980);
#12368=VERTEX_POINT('',#43985);
#12369=VERTEX_POINT('',#43986);
#12370=VERTEX_POINT('',#43991);
#12371=VERTEX_POINT('',#43992);
#12372=VERTEX_POINT('',#43997);
#12373=VERTEX_POINT('',#44002);
#15370=EDGE_CURVE('',#12235,#12236,#7402,.T.);
#15371=EDGE_CURVE('',#12236,#12237,#2238,.T.);
#15372=EDGE_CURVE('',#12237,#12238,#7403,.T.);
#15373=EDGE_CURVE('',#12238,#12235,#2239,.T.);
#15374=EDGE_CURVE('',#12239,#12240,#7404,.T.);
#15375=EDGE_CURVE('',#12240,#12236,#7405,.T.);
#15376=EDGE_CURVE('',#12235,#12239,#7406,.T.);
#15377=EDGE_CURVE('',#12241,#12242,#7407,.T.);
#15378=EDGE_CURVE('',#12242,#12240,#2240,.T.);
#15379=EDGE_CURVE('',#12239,#12241,#2241,.T.);
#15380=EDGE_CURVE('',#12243,#12244,#7408,.T.);
#15381=EDGE_CURVE('',#12244,#12242,#7409,.T.);
#15382=EDGE_CURVE('',#12241,#12243,#7410,.T.);
#15383=EDGE_CURVE('',#12245,#12246,#7411,.T.);
#15384=EDGE_CURVE('',#12246,#12244,#2242,.T.);
#15385=EDGE_CURVE('',#12243,#12245,#2243,.T.);
#15386=EDGE_CURVE('',#12247,#12248,#7412,.T.);
#15387=EDGE_CURVE('',#12248,#12246,#7413,.T.);
#15388=EDGE_CURVE('',#12245,#12247,#7414,.T.);
#15389=EDGE_CURVE('',#12249,#12250,#7415,.T.);
#15390=EDGE_CURVE('',#12250,#12248,#2244,.T.);
#15391=EDGE_CURVE('',#12247,#12249,#2245,.T.);
#15392=EDGE_CURVE('',#12237,#12250,#7416,.T.);
#15393=EDGE_CURVE('',#12249,#12238,#7417,.T.);
#15394=EDGE_CURVE('',#12248,#12251,#7418,.T.);
#15395=EDGE_CURVE('',#12252,#12251,#7419,.T.);
#15396=EDGE_CURVE('',#12246,#12252,#7420,.T.);
#15397=EDGE_CURVE('',#12250,#12253,#7421,.T.);
#15398=EDGE_CURVE('',#12251,#12253,#2246,.T.);
#15399=EDGE_CURVE('',#12254,#12237,#7422,.T.);
#15400=EDGE_CURVE('',#12253,#12254,#7423,.T.);
#15401=EDGE_CURVE('',#12236,#12255,#7424,.T.);
#15402=EDGE_CURVE('',#12254,#12255,#2247,.T.);
#15403=EDGE_CURVE('',#12256,#12256,#2248,.T.);
#15404=EDGE_CURVE('',#12257,#12257,#2249,.T.);
#15405=EDGE_CURVE('',#12258,#12258,#2250,.T.);
#15406=EDGE_CURVE('',#12259,#12260,#7425,.F.);
#15407=EDGE_CURVE('',#12260,#12261,#7426,.T.);
#15408=EDGE_CURVE('',#12261,#12262,#7427,.F.);
#15409=EDGE_CURVE('',#12262,#12259,#7428,.T.);
#15410=EDGE_CURVE('',#12260,#12263,#2251,.T.);
#15411=EDGE_CURVE('',#12264,#12263,#7429,.T.);
#15412=EDGE_CURVE('',#12261,#12264,#2252,.T.);
#15413=EDGE_CURVE('',#12265,#12264,#7430,.F.);
#15414=EDGE_CURVE('',#12263,#12266,#7431,.F.);
#15415=EDGE_CURVE('',#12266,#12265,#7432,.T.);
#15416=EDGE_CURVE('',#12267,#12253,#7433,.T.);
#15417=EDGE_CURVE('',#12254,#12268,#7434,.T.);
#15418=EDGE_CURVE('',#12268,#12267,#7435,.T.);
#15419=EDGE_CURVE('',#12269,#12251,#7436,.T.);
#15420=EDGE_CURVE('',#12267,#12269,#2253,.T.);
#15421=EDGE_CURVE('',#12270,#12252,#7437,.T.);
#15422=EDGE_CURVE('',#12269,#12270,#7438,.T.);
#15423=EDGE_CURVE('',#12271,#12272,#7439,.T.);
#15424=EDGE_CURVE('',#12272,#12252,#2254,.T.);
#15425=EDGE_CURVE('',#12270,#12271,#2255,.T.);
#15426=EDGE_CURVE('',#12273,#12274,#7440,.T.);
#15427=EDGE_CURVE('',#12274,#12272,#7441,.T.);
#15428=EDGE_CURVE('',#12271,#12273,#7442,.T.);
#15429=EDGE_CURVE('',#12275,#12276,#7443,.T.);
#15430=EDGE_CURVE('',#12276,#12274,#2256,.T.);
#15431=EDGE_CURVE('',#12273,#12275,#2257,.T.);
#15432=EDGE_CURVE('',#12277,#12255,#7444,.T.);
#15433=EDGE_CURVE('',#12255,#12276,#7445,.T.);
#15434=EDGE_CURVE('',#12275,#12277,#7446,.T.);
#15435=EDGE_CURVE('',#12277,#12268,#2258,.T.);
#15436=EDGE_CURVE('',#12270,#12278,#7447,.T.);
#15437=EDGE_CURVE('',#12279,#12278,#2259,.T.);
#15438=EDGE_CURVE('',#12279,#12271,#7448,.T.);
#15439=EDGE_CURVE('',#12280,#12269,#7449,.T.);
#15440=EDGE_CURVE('',#12278,#12280,#7450,.T.);
#15441=EDGE_CURVE('',#12267,#12281,#7451,.T.);
#15442=EDGE_CURVE('',#12280,#12281,#2260,.T.);
#15443=EDGE_CURVE('',#12282,#12268,#7452,.T.);
#15444=EDGE_CURVE('',#12281,#12282,#7453,.T.);
#15445=EDGE_CURVE('',#12283,#12283,#2261,.T.);
#15446=EDGE_CURVE('',#12242,#12274,#7454,.T.);
#15447=EDGE_CURVE('',#12240,#12276,#7455,.T.);
#15448=EDGE_CURVE('',#12284,#12285,#7456,.T.);
#15449=EDGE_CURVE('',#12285,#12286,#7457,.T.);
#15450=EDGE_CURVE('',#12286,#12287,#7458,.T.);
#15451=EDGE_CURVE('',#12287,#12284,#7459,.T.);
#15452=EDGE_CURVE('',#12288,#12289,#7460,.T.);
#15453=EDGE_CURVE('',#12289,#12287,#2262,.T.);
#15454=EDGE_CURVE('',#12286,#12288,#2263,.T.);
#15455=EDGE_CURVE('',#12290,#12291,#7461,.T.);
#15456=EDGE_CURVE('',#12291,#12289,#7462,.T.);
#15457=EDGE_CURVE('',#12288,#12290,#7463,.T.);
#15458=EDGE_CURVE('',#12292,#12293,#7464,.T.);
#15459=EDGE_CURVE('',#12293,#12291,#2264,.T.);
#15460=EDGE_CURVE('',#12290,#12292,#2265,.T.);
#15461=EDGE_CURVE('',#12294,#12295,#7465,.T.);
#15462=EDGE_CURVE('',#12295,#12293,#7466,.T.);
#15463=EDGE_CURVE('',#12292,#12294,#7467,.T.);
#15464=EDGE_CURVE('',#12296,#12294,#7468,.T.);
#15465=EDGE_CURVE('',#12297,#12296,#2266,.T.);
#15466=EDGE_CURVE('',#12295,#12297,#7469,.T.);
#15467=EDGE_CURVE('',#12285,#12298,#7470,.T.);
#15468=EDGE_CURVE('',#12296,#12298,#7471,.T.);
#15469=EDGE_CURVE('',#12299,#12300,#7472,.F.);
#15470=EDGE_CURVE('',#12300,#12301,#7473,.T.);
#15471=EDGE_CURVE('',#12301,#12302,#7474,.T.);
#15472=EDGE_CURVE('',#12302,#12299,#7475,.T.);
#15473=EDGE_CURVE('',#12303,#12304,#7476,.T.);
#15474=EDGE_CURVE('',#12304,#12302,#2267,.T.);
#15475=EDGE_CURVE('',#12301,#12303,#2268,.T.);
#15476=EDGE_CURVE('',#12305,#12306,#7477,.T.);
#15477=EDGE_CURVE('',#12306,#12304,#7478,.T.);
#15478=EDGE_CURVE('',#12303,#12305,#7479,.T.);
#15479=EDGE_CURVE('',#12307,#12308,#7480,.T.);
#15480=EDGE_CURVE('',#12308,#12306,#2269,.T.);
#15481=EDGE_CURVE('',#12305,#12307,#2270,.T.);
#15482=EDGE_CURVE('',#12309,#12310,#7481,.F.);
#15483=EDGE_CURVE('',#12310,#12308,#7482,.T.);
#15484=EDGE_CURVE('',#12307,#12309,#7483,.T.);
#15485=EDGE_CURVE('',#12309,#12300,#7484,.T.);
#15486=EDGE_CURVE('',#12311,#12311,#2271,.T.);
#15487=EDGE_CURVE('',#12312,#12313,#7485,.F.);
#15488=EDGE_CURVE('',#12313,#12314,#7486,.T.);
#15489=EDGE_CURVE('',#12314,#12315,#7487,.T.);
#15490=EDGE_CURVE('',#12315,#12312,#7488,.T.);
#15491=EDGE_CURVE('',#12316,#12317,#7489,.T.);
#15492=EDGE_CURVE('',#12317,#12315,#2272,.T.);
#15493=EDGE_CURVE('',#12314,#12316,#2273,.T.);
#15494=EDGE_CURVE('',#12318,#12319,#7490,.T.);
#15495=EDGE_CURVE('',#12319,#12317,#7491,.T.);
#15496=EDGE_CURVE('',#12316,#12318,#7492,.T.);
#15497=EDGE_CURVE('',#12320,#12321,#7493,.T.);
#15498=EDGE_CURVE('',#12321,#12319,#2274,.T.);
#15499=EDGE_CURVE('',#12318,#12320,#2275,.T.);
#15500=EDGE_CURVE('',#12322,#12323,#7494,.F.);
#15501=EDGE_CURVE('',#12323,#12321,#7495,.T.);
#15502=EDGE_CURVE('',#12320,#12322,#7496,.T.);
#15503=EDGE_CURVE('',#12322,#12313,#7497,.T.);
#15504=EDGE_CURVE('',#12324,#12324,#2276,.T.);
#15505=EDGE_CURVE('',#12325,#12326,#7498,.T.);
#15506=EDGE_CURVE('',#12326,#12327,#7499,.T.);
#15507=EDGE_CURVE('',#12327,#12328,#7500,.T.);
#15508=EDGE_CURVE('',#12328,#12325,#7501,.T.);
#15509=EDGE_CURVE('',#12329,#12330,#7502,.T.);
#15510=EDGE_CURVE('',#12330,#12328,#2277,.T.);
#15511=EDGE_CURVE('',#12327,#12329,#2278,.T.);
#15512=EDGE_CURVE('',#12331,#12332,#7503,.T.);
#15513=EDGE_CURVE('',#12332,#12330,#7504,.T.);
#15514=EDGE_CURVE('',#12329,#12331,#7505,.T.);
#15515=EDGE_CURVE('',#12333,#12334,#7506,.T.);
#15516=EDGE_CURVE('',#12334,#12332,#2279,.T.);
#15517=EDGE_CURVE('',#12331,#12333,#2280,.T.);
#15518=EDGE_CURVE('',#12335,#12336,#7507,.T.);
#15519=EDGE_CURVE('',#12336,#12334,#7508,.T.);
#15520=EDGE_CURVE('',#12333,#12335,#7509,.T.);
#15521=EDGE_CURVE('',#12337,#12323,#7510,.T.);
#15522=EDGE_CURVE('',#12337,#12325,#7511,.T.);
#15523=EDGE_CURVE('',#12321,#12328,#7512,.T.);
#15524=EDGE_CURVE('',#12330,#12319,#7513,.T.);
#15525=EDGE_CURVE('',#12317,#12332,#7514,.T.);
#15526=EDGE_CURVE('',#12334,#12315,#7515,.T.);
#15527=EDGE_CURVE('',#12336,#12338,#7516,.T.);
#15528=EDGE_CURVE('',#12312,#12338,#7517,.T.);
#15529=EDGE_CURVE('',#12339,#12335,#7518,.T.);
#15530=EDGE_CURVE('',#12338,#12339,#2281,.T.);
#15531=EDGE_CURVE('',#12340,#12340,#2282,.T.);
#15532=EDGE_CURVE('',#12340,#12341,#7519,.T.);
#15533=EDGE_CURVE('',#12341,#12341,#2283,.T.);
#15534=EDGE_CURVE('',#12342,#12342,#2284,.T.);
#15535=EDGE_CURVE('',#12341,#12258,#7520,.T.);
#15536=EDGE_CURVE('',#12342,#12343,#7521,.T.);
#15537=EDGE_CURVE('',#12343,#12343,#2285,.T.);
#15538=EDGE_CURVE('',#12344,#12344,#2286,.T.);
#15539=EDGE_CURVE('',#12344,#12343,#7522,.T.);
#15540=EDGE_CURVE('',#12283,#12345,#7523,.T.);
#15541=EDGE_CURVE('',#12345,#12345,#2287,.T.);
#15542=EDGE_CURVE('',#12345,#12346,#7524,.T.);
#15543=EDGE_CURVE('',#12346,#12346,#2288,.T.);
#15544=EDGE_CURVE('',#12346,#12347,#7525,.T.);
#15545=EDGE_CURVE('',#12348,#12344,#7526,.T.);
#15546=EDGE_CURVE('',#12311,#12324,#7527,.T.);
#15547=EDGE_CURVE('',#12293,#12302,#7528,.T.);
#15548=EDGE_CURVE('',#12304,#12291,#7529,.T.);
#15549=EDGE_CURVE('',#12289,#12306,#7530,.T.);
#15550=EDGE_CURVE('',#12308,#12287,#7531,.T.);
#15551=EDGE_CURVE('',#12349,#12284,#7532,.T.);
#15552=EDGE_CURVE('',#12298,#12349,#2289,.T.);
#15553=EDGE_CURVE('',#12349,#12310,#7533,.T.);
#15554=EDGE_CURVE('',#12299,#12297,#7534,.T.);
#15555=EDGE_CURVE('',#12296,#12298,#2290,.T.);
#15556=EDGE_CURVE('',#12350,#12337,#2291,.T.);
#15557=EDGE_CURVE('',#12326,#12350,#7535,.T.);
#15558=EDGE_CURVE('',#12339,#12350,#7536,.T.);
#15559=EDGE_CURVE('',#12339,#12350,#2292,.T.);
#15560=EDGE_CURVE('',#12351,#12297,#2293,.T.);
#15561=EDGE_CURVE('',#12337,#12351,#2294,.T.);
#15562=EDGE_CURVE('',#12349,#12338,#2295,.T.);
#15563=EDGE_CURVE('',#12351,#12352,#7537,.T.);
#15564=EDGE_CURVE('',#12352,#12352,#2296,.T.);
#15565=EDGE_CURVE('',#12352,#12257,#7538,.T.);
#15566=EDGE_CURVE('',#12353,#12353,#2297,.T.);
#15567=EDGE_CURVE('',#12353,#12354,#7539,.T.);
#15568=EDGE_CURVE('',#12354,#12354,#2298,.T.);
#15569=EDGE_CURVE('',#12355,#12355,#2299,.T.);
#15570=EDGE_CURVE('',#12355,#12354,#7540,.T.);
#15571=EDGE_CURVE('',#12356,#12356,#2300,.T.);
#15572=EDGE_CURVE('',#12266,#12259,#2301,.T.);
#15573=EDGE_CURVE('',#12262,#12265,#2302,.T.);
#15574=EDGE_CURVE('',#12357,#12358,#2303,.T.);
#15575=EDGE_CURVE('',#12358,#12256,#2304,.T.);
#15576=EDGE_CURVE('',#12358,#12357,#2305,.T.);
#15577=EDGE_CURVE('',#12359,#12359,#2306,.T.);
#15578=EDGE_CURVE('',#12359,#12357,#7541,.T.);
#15579=EDGE_CURVE('',#12360,#12360,#2307,.T.);
#15580=EDGE_CURVE('',#12361,#12361,#2308,.T.);
#15581=EDGE_CURVE('',#12361,#12360,#7542,.T.);
#15582=EDGE_CURVE('',#12362,#12362,#2309,.T.);
#15583=EDGE_CURVE('',#12362,#12361,#7543,.T.);
#15584=EDGE_CURVE('',#12356,#12362,#7544,.T.);
#15585=EDGE_CURVE('',#12363,#12278,#7545,.T.);
#15586=EDGE_CURVE('',#12280,#12364,#7546,.T.);
#15587=EDGE_CURVE('',#12364,#12363,#7547,.T.);
#15588=EDGE_CURVE('',#12365,#12279,#7548,.T.);
#15589=EDGE_CURVE('',#12363,#12365,#2310,.T.);
#15590=EDGE_CURVE('',#12366,#12367,#7549,.T.);
#15591=EDGE_CURVE('',#12367,#12279,#7550,.T.);
#15592=EDGE_CURVE('',#12365,#12366,#7551,.T.);
#15593=EDGE_CURVE('',#12368,#12369,#7552,.T.);
#15594=EDGE_CURVE('',#12369,#12367,#2311,.T.);
#15595=EDGE_CURVE('',#12366,#12368,#2312,.T.);
#15596=EDGE_CURVE('',#12370,#12371,#7553,.T.);
#15597=EDGE_CURVE('',#12371,#12369,#7554,.T.);
#15598=EDGE_CURVE('',#12368,#12370,#7555,.T.);
#15599=EDGE_CURVE('',#12372,#12282,#7556,.T.);
#15600=EDGE_CURVE('',#12282,#12371,#2313,.T.);
#15601=EDGE_CURVE('',#12370,#12372,#2314,.T.);
#15602=EDGE_CURVE('',#12373,#12281,#7557,.T.);
#15603=EDGE_CURVE('',#12372,#12373,#7558,.T.);
#15604=EDGE_CURVE('',#12373,#12364,#2315,.T.);
#15605=EDGE_CURVE('',#12277,#12371,#7559,.T.);
#15606=EDGE_CURVE('',#12244,#12272,#7560,.T.);
#15607=EDGE_CURVE('',#12369,#12275,#7561,.T.);
#15608=EDGE_CURVE('',#12273,#12367,#7562,.T.);
#20973=ORIENTED_EDGE('',*,*,#15370,.T.);
#20974=ORIENTED_EDGE('',*,*,#15371,.T.);
#20975=ORIENTED_EDGE('',*,*,#15372,.T.);
#20976=ORIENTED_EDGE('',*,*,#15373,.T.);
#20977=ORIENTED_EDGE('',*,*,#15374,.T.);
#20978=ORIENTED_EDGE('',*,*,#15375,.T.);
#20979=ORIENTED_EDGE('',*,*,#15370,.F.);
#20980=ORIENTED_EDGE('',*,*,#15376,.T.);
#20981=ORIENTED_EDGE('',*,*,#15377,.T.);
#20982=ORIENTED_EDGE('',*,*,#15378,.T.);
#20983=ORIENTED_EDGE('',*,*,#15374,.F.);
#20984=ORIENTED_EDGE('',*,*,#15379,.T.);
#20985=ORIENTED_EDGE('',*,*,#15380,.T.);
#20986=ORIENTED_EDGE('',*,*,#15381,.T.);
#20987=ORIENTED_EDGE('',*,*,#15377,.F.);
#20988=ORIENTED_EDGE('',*,*,#15382,.T.);
#20989=ORIENTED_EDGE('',*,*,#15383,.T.);
#20990=ORIENTED_EDGE('',*,*,#15384,.T.);
#20991=ORIENTED_EDGE('',*,*,#15380,.F.);
#20992=ORIENTED_EDGE('',*,*,#15385,.T.);
#20993=ORIENTED_EDGE('',*,*,#15386,.T.);
#20994=ORIENTED_EDGE('',*,*,#15387,.T.);
#20995=ORIENTED_EDGE('',*,*,#15383,.F.);
#20996=ORIENTED_EDGE('',*,*,#15388,.T.);
#20997=ORIENTED_EDGE('',*,*,#15389,.T.);
#20998=ORIENTED_EDGE('',*,*,#15390,.T.);
#20999=ORIENTED_EDGE('',*,*,#15386,.F.);
#21000=ORIENTED_EDGE('',*,*,#15391,.T.);
#21001=ORIENTED_EDGE('',*,*,#15372,.F.);
#21002=ORIENTED_EDGE('',*,*,#15392,.T.);
#21003=ORIENTED_EDGE('',*,*,#15389,.F.);
#21004=ORIENTED_EDGE('',*,*,#15393,.T.);
#21005=ORIENTED_EDGE('',*,*,#15387,.F.);
#21006=ORIENTED_EDGE('',*,*,#15394,.T.);
#21007=ORIENTED_EDGE('',*,*,#15395,.F.);
#21008=ORIENTED_EDGE('',*,*,#15396,.F.);
#21009=ORIENTED_EDGE('',*,*,#15390,.F.);
#21010=ORIENTED_EDGE('',*,*,#15397,.T.);
#21011=ORIENTED_EDGE('',*,*,#15398,.F.);
#21012=ORIENTED_EDGE('',*,*,#15394,.F.);
#21013=ORIENTED_EDGE('',*,*,#15392,.F.);
#21014=ORIENTED_EDGE('',*,*,#15399,.F.);
#21015=ORIENTED_EDGE('',*,*,#15400,.F.);
#21016=ORIENTED_EDGE('',*,*,#15397,.F.);
#21017=ORIENTED_EDGE('',*,*,#15371,.F.);
#21018=ORIENTED_EDGE('',*,*,#15401,.T.);
#21019=ORIENTED_EDGE('',*,*,#15402,.F.);
#21020=ORIENTED_EDGE('',*,*,#15399,.T.);
#21021=ORIENTED_EDGE('',*,*,#15373,.F.);
#21022=ORIENTED_EDGE('',*,*,#15393,.F.);
#21023=ORIENTED_EDGE('',*,*,#15391,.F.);
#21024=ORIENTED_EDGE('',*,*,#15388,.F.);
#21025=ORIENTED_EDGE('',*,*,#15385,.F.);
#21026=ORIENTED_EDGE('',*,*,#15382,.F.);
#21027=ORIENTED_EDGE('',*,*,#15379,.F.);
#21028=ORIENTED_EDGE('',*,*,#15376,.F.);
#21029=ORIENTED_EDGE('',*,*,#15403,.F.);
#21030=ORIENTED_EDGE('',*,*,#15404,.T.);
#21031=ORIENTED_EDGE('',*,*,#15405,.T.);
#21032=ORIENTED_EDGE('',*,*,#15406,.T.);
#21033=ORIENTED_EDGE('',*,*,#15407,.T.);
#21034=ORIENTED_EDGE('',*,*,#15408,.T.);
#21035=ORIENTED_EDGE('',*,*,#15409,.T.);
#21036=ORIENTED_EDGE('',*,*,#15407,.F.);
#21037=ORIENTED_EDGE('',*,*,#15410,.T.);
#21038=ORIENTED_EDGE('',*,*,#15411,.F.);
#21039=ORIENTED_EDGE('',*,*,#15412,.F.);
#21040=ORIENTED_EDGE('',*,*,#15413,.T.);
#21041=ORIENTED_EDGE('',*,*,#15411,.T.);
#21042=ORIENTED_EDGE('',*,*,#15414,.T.);
#21043=ORIENTED_EDGE('',*,*,#15415,.T.);
#21044=ORIENTED_EDGE('',*,*,#15416,.T.);
#21045=ORIENTED_EDGE('',*,*,#15400,.T.);
#21046=ORIENTED_EDGE('',*,*,#15417,.T.);
#21047=ORIENTED_EDGE('',*,*,#15418,.T.);
#21048=ORIENTED_EDGE('',*,*,#15419,.T.);
#21049=ORIENTED_EDGE('',*,*,#15398,.T.);
#21050=ORIENTED_EDGE('',*,*,#15416,.F.);
#21051=ORIENTED_EDGE('',*,*,#15420,.T.);
#21052=ORIENTED_EDGE('',*,*,#15421,.T.);
#21053=ORIENTED_EDGE('',*,*,#15395,.T.);
#21054=ORIENTED_EDGE('',*,*,#15419,.F.);
#21055=ORIENTED_EDGE('',*,*,#15422,.T.);
#21056=ORIENTED_EDGE('',*,*,#15423,.T.);
#21057=ORIENTED_EDGE('',*,*,#15424,.T.);
#21058=ORIENTED_EDGE('',*,*,#15421,.F.);
#21059=ORIENTED_EDGE('',*,*,#15425,.T.);
#21060=ORIENTED_EDGE('',*,*,#15426,.T.);
#21061=ORIENTED_EDGE('',*,*,#15427,.T.);
#21062=ORIENTED_EDGE('',*,*,#15423,.F.);
#21063=ORIENTED_EDGE('',*,*,#15428,.T.);
#21064=ORIENTED_EDGE('',*,*,#15429,.T.);
#21065=ORIENTED_EDGE('',*,*,#15430,.T.);
#21066=ORIENTED_EDGE('',*,*,#15426,.F.);
#21067=ORIENTED_EDGE('',*,*,#15431,.T.);
#21068=ORIENTED_EDGE('',*,*,#15432,.T.);
#21069=ORIENTED_EDGE('',*,*,#15433,.T.);
#21070=ORIENTED_EDGE('',*,*,#15429,.F.);
#21071=ORIENTED_EDGE('',*,*,#15434,.T.);
#21072=ORIENTED_EDGE('',*,*,#15417,.F.);
#21073=ORIENTED_EDGE('',*,*,#15402,.T.);
#21074=ORIENTED_EDGE('',*,*,#15432,.F.);
#21075=ORIENTED_EDGE('',*,*,#15435,.T.);
#21076=ORIENTED_EDGE('',*,*,#15425,.F.);
#21077=ORIENTED_EDGE('',*,*,#15436,.T.);
#21078=ORIENTED_EDGE('',*,*,#15437,.F.);
#21079=ORIENTED_EDGE('',*,*,#15438,.T.);
#21080=ORIENTED_EDGE('',*,*,#15422,.F.);
#21081=ORIENTED_EDGE('',*,*,#15439,.F.);
#21082=ORIENTED_EDGE('',*,*,#15440,.F.);
#21083=ORIENTED_EDGE('',*,*,#15436,.F.);
#21084=ORIENTED_EDGE('',*,*,#15420,.F.);
#21085=ORIENTED_EDGE('',*,*,#15441,.T.);
#21086=ORIENTED_EDGE('',*,*,#15442,.F.);
#21087=ORIENTED_EDGE('',*,*,#15439,.T.);
#21088=ORIENTED_EDGE('',*,*,#15418,.F.);
#21089=ORIENTED_EDGE('',*,*,#15443,.F.);
#21090=ORIENTED_EDGE('',*,*,#15444,.F.);
#21091=ORIENTED_EDGE('',*,*,#15441,.F.);
#21092=ORIENTED_EDGE('',*,*,#15445,.F.);
#21093=ORIENTED_EDGE('',*,*,#15378,.F.);
#21094=ORIENTED_EDGE('',*,*,#15446,.T.);
#21095=ORIENTED_EDGE('',*,*,#15430,.F.);
#21096=ORIENTED_EDGE('',*,*,#15447,.F.);
#21097=ORIENTED_EDGE('',*,*,#15375,.F.);
#21098=ORIENTED_EDGE('',*,*,#15447,.T.);
#21099=ORIENTED_EDGE('',*,*,#15433,.F.);
#21100=ORIENTED_EDGE('',*,*,#15401,.F.);
#21101=ORIENTED_EDGE('',*,*,#15448,.T.);
#21102=ORIENTED_EDGE('',*,*,#15449,.T.);
#21103=ORIENTED_EDGE('',*,*,#15450,.T.);
#21104=ORIENTED_EDGE('',*,*,#15451,.T.);
#21105=ORIENTED_EDGE('',*,*,#15452,.T.);
#21106=ORIENTED_EDGE('',*,*,#15453,.T.);
#21107=ORIENTED_EDGE('',*,*,#15450,.F.);
#21108=ORIENTED_EDGE('',*,*,#15454,.T.);
#21109=ORIENTED_EDGE('',*,*,#15455,.T.);
#21110=ORIENTED_EDGE('',*,*,#15456,.T.);
#21111=ORIENTED_EDGE('',*,*,#15452,.F.);
#21112=ORIENTED_EDGE('',*,*,#15457,.T.);
#21113=ORIENTED_EDGE('',*,*,#15458,.T.);
#21114=ORIENTED_EDGE('',*,*,#15459,.T.);
#21115=ORIENTED_EDGE('',*,*,#15455,.F.);
#21116=ORIENTED_EDGE('',*,*,#15460,.T.);
#21117=ORIENTED_EDGE('',*,*,#15461,.T.);
#21118=ORIENTED_EDGE('',*,*,#15462,.T.);
#21119=ORIENTED_EDGE('',*,*,#15458,.F.);
#21120=ORIENTED_EDGE('',*,*,#15463,.T.);
#21121=ORIENTED_EDGE('',*,*,#15461,.F.);
#21122=ORIENTED_EDGE('',*,*,#15464,.F.);
#21123=ORIENTED_EDGE('',*,*,#15465,.F.);
#21124=ORIENTED_EDGE('',*,*,#15466,.F.);
#21125=ORIENTED_EDGE('',*,*,#15463,.F.);
#21126=ORIENTED_EDGE('',*,*,#15460,.F.);
#21127=ORIENTED_EDGE('',*,*,#15457,.F.);
#21128=ORIENTED_EDGE('',*,*,#15454,.F.);
#21129=ORIENTED_EDGE('',*,*,#15449,.F.);
#21130=ORIENTED_EDGE('',*,*,#15467,.T.);
#21131=ORIENTED_EDGE('',*,*,#15468,.F.);
#21132=ORIENTED_EDGE('',*,*,#15464,.T.);
#21133=ORIENTED_EDGE('',*,*,#15469,.T.);
#21134=ORIENTED_EDGE('',*,*,#15470,.T.);
#21135=ORIENTED_EDGE('',*,*,#15471,.T.);
#21136=ORIENTED_EDGE('',*,*,#15472,.T.);
#21137=ORIENTED_EDGE('',*,*,#15473,.T.);
#21138=ORIENTED_EDGE('',*,*,#15474,.T.);
#21139=ORIENTED_EDGE('',*,*,#15471,.F.);
#21140=ORIENTED_EDGE('',*,*,#15475,.T.);
#21141=ORIENTED_EDGE('',*,*,#15476,.T.);
#21142=ORIENTED_EDGE('',*,*,#15477,.T.);
#21143=ORIENTED_EDGE('',*,*,#15473,.F.);
#21144=ORIENTED_EDGE('',*,*,#15478,.T.);
#21145=ORIENTED_EDGE('',*,*,#15479,.T.);
#21146=ORIENTED_EDGE('',*,*,#15480,.T.);
#21147=ORIENTED_EDGE('',*,*,#15476,.F.);
#21148=ORIENTED_EDGE('',*,*,#15481,.T.);
#21149=ORIENTED_EDGE('',*,*,#15482,.T.);
#21150=ORIENTED_EDGE('',*,*,#15483,.T.);
#21151=ORIENTED_EDGE('',*,*,#15479,.F.);
#21152=ORIENTED_EDGE('',*,*,#15484,.T.);
#21153=ORIENTED_EDGE('',*,*,#15484,.F.);
#21154=ORIENTED_EDGE('',*,*,#15481,.F.);
#21155=ORIENTED_EDGE('',*,*,#15478,.F.);
#21156=ORIENTED_EDGE('',*,*,#15475,.F.);
#21157=ORIENTED_EDGE('',*,*,#15470,.F.);
#21158=ORIENTED_EDGE('',*,*,#15485,.F.);
#21159=ORIENTED_EDGE('',*,*,#15486,.T.);
#21160=ORIENTED_EDGE('',*,*,#15487,.T.);
#21161=ORIENTED_EDGE('',*,*,#15488,.T.);
#21162=ORIENTED_EDGE('',*,*,#15489,.T.);
#21163=ORIENTED_EDGE('',*,*,#15490,.T.);
#21164=ORIENTED_EDGE('',*,*,#15491,.T.);
#21165=ORIENTED_EDGE('',*,*,#15492,.T.);
#21166=ORIENTED_EDGE('',*,*,#15489,.F.);
#21167=ORIENTED_EDGE('',*,*,#15493,.T.);
#21168=ORIENTED_EDGE('',*,*,#15494,.T.);
#21169=ORIENTED_EDGE('',*,*,#15495,.T.);
#21170=ORIENTED_EDGE('',*,*,#15491,.F.);
#21171=ORIENTED_EDGE('',*,*,#15496,.T.);
#21172=ORIENTED_EDGE('',*,*,#15497,.T.);
#21173=ORIENTED_EDGE('',*,*,#15498,.T.);
#21174=ORIENTED_EDGE('',*,*,#15494,.F.);
#21175=ORIENTED_EDGE('',*,*,#15499,.T.);
#21176=ORIENTED_EDGE('',*,*,#15500,.T.);
#21177=ORIENTED_EDGE('',*,*,#15501,.T.);
#21178=ORIENTED_EDGE('',*,*,#15497,.F.);
#21179=ORIENTED_EDGE('',*,*,#15502,.T.);
#21180=ORIENTED_EDGE('',*,*,#15502,.F.);
#21181=ORIENTED_EDGE('',*,*,#15499,.F.);
#21182=ORIENTED_EDGE('',*,*,#15496,.F.);
#21183=ORIENTED_EDGE('',*,*,#15493,.F.);
#21184=ORIENTED_EDGE('',*,*,#15488,.F.);
#21185=ORIENTED_EDGE('',*,*,#15503,.F.);
#21186=ORIENTED_EDGE('',*,*,#15504,.T.);
#21187=ORIENTED_EDGE('',*,*,#15505,.T.);
#21188=ORIENTED_EDGE('',*,*,#15506,.T.);
#21189=ORIENTED_EDGE('',*,*,#15507,.T.);
#21190=ORIENTED_EDGE('',*,*,#15508,.T.);
#21191=ORIENTED_EDGE('',*,*,#15509,.T.);
#21192=ORIENTED_EDGE('',*,*,#15510,.T.);
#21193=ORIENTED_EDGE('',*,*,#15507,.F.);
#21194=ORIENTED_EDGE('',*,*,#15511,.T.);
#21195=ORIENTED_EDGE('',*,*,#15512,.T.);
#21196=ORIENTED_EDGE('',*,*,#15513,.T.);
#21197=ORIENTED_EDGE('',*,*,#15509,.F.);
#21198=ORIENTED_EDGE('',*,*,#15514,.T.);
#21199=ORIENTED_EDGE('',*,*,#15515,.T.);
#21200=ORIENTED_EDGE('',*,*,#15516,.T.);
#21201=ORIENTED_EDGE('',*,*,#15512,.F.);
#21202=ORIENTED_EDGE('',*,*,#15517,.T.);
#21203=ORIENTED_EDGE('',*,*,#15518,.T.);
#21204=ORIENTED_EDGE('',*,*,#15519,.T.);
#21205=ORIENTED_EDGE('',*,*,#15515,.F.);
#21206=ORIENTED_EDGE('',*,*,#15520,.T.);
#21207=ORIENTED_EDGE('',*,*,#15501,.F.);
#21208=ORIENTED_EDGE('',*,*,#15521,.F.);
#21209=ORIENTED_EDGE('',*,*,#15522,.T.);
#21210=ORIENTED_EDGE('',*,*,#15508,.F.);
#21211=ORIENTED_EDGE('',*,*,#15523,.F.);
#21212=ORIENTED_EDGE('',*,*,#15498,.F.);
#21213=ORIENTED_EDGE('',*,*,#15523,.T.);
#21214=ORIENTED_EDGE('',*,*,#15510,.F.);
#21215=ORIENTED_EDGE('',*,*,#15524,.T.);
#21216=ORIENTED_EDGE('',*,*,#15495,.F.);
#21217=ORIENTED_EDGE('',*,*,#15524,.F.);
#21218=ORIENTED_EDGE('',*,*,#15513,.F.);
#21219=ORIENTED_EDGE('',*,*,#15525,.F.);
#21220=ORIENTED_EDGE('',*,*,#15492,.F.);
#21221=ORIENTED_EDGE('',*,*,#15525,.T.);
#21222=ORIENTED_EDGE('',*,*,#15516,.F.);
#21223=ORIENTED_EDGE('',*,*,#15526,.T.);
#21224=ORIENTED_EDGE('',*,*,#15490,.F.);
#21225=ORIENTED_EDGE('',*,*,#15526,.F.);
#21226=ORIENTED_EDGE('',*,*,#15519,.F.);
#21227=ORIENTED_EDGE('',*,*,#15527,.T.);
#21228=ORIENTED_EDGE('',*,*,#15528,.F.);
#21229=ORIENTED_EDGE('',*,*,#15518,.F.);
#21230=ORIENTED_EDGE('',*,*,#15529,.F.);
#21231=ORIENTED_EDGE('',*,*,#15530,.F.);
#21232=ORIENTED_EDGE('',*,*,#15527,.F.);
#21233=ORIENTED_EDGE('',*,*,#15531,.T.);
#21234=ORIENTED_EDGE('',*,*,#15532,.T.);
#21235=ORIENTED_EDGE('',*,*,#15533,.T.);
#21236=ORIENTED_EDGE('',*,*,#15532,.F.);
#21237=ORIENTED_EDGE('',*,*,#15531,.F.);
#21238=ORIENTED_EDGE('',*,*,#15534,.F.);
#21239=ORIENTED_EDGE('',*,*,#15533,.F.);
#21240=ORIENTED_EDGE('',*,*,#15535,.T.);
#21241=ORIENTED_EDGE('',*,*,#15405,.F.);
#21242=ORIENTED_EDGE('',*,*,#15535,.F.);
#21243=ORIENTED_EDGE('',*,*,#15534,.T.);
#21244=ORIENTED_EDGE('',*,*,#15536,.T.);
#21245=ORIENTED_EDGE('',*,*,#15537,.T.);
#21246=ORIENTED_EDGE('',*,*,#15536,.F.);
#21247=ORIENTED_EDGE('',*,*,#15538,.F.);
#21248=ORIENTED_EDGE('',*,*,#15539,.T.);
#21249=ORIENTED_EDGE('',*,*,#15537,.F.);
#21250=ORIENTED_EDGE('',*,*,#15539,.F.);
#21251=ORIENTED_EDGE('',*,*,#15445,.T.);
#21252=ORIENTED_EDGE('',*,*,#15540,.T.);
#21253=ORIENTED_EDGE('',*,*,#15541,.T.);
#21254=ORIENTED_EDGE('',*,*,#15540,.F.);
#21255=ORIENTED_EDGE('',*,*,#15541,.F.);
#21256=ORIENTED_EDGE('',*,*,#15542,.T.);
#21257=ORIENTED_EDGE('',*,*,#15543,.T.);
#21258=ORIENTED_EDGE('',*,*,#15542,.F.);
#21259=ORIENTED_EDGE('',*,*,#15543,.F.);
#21260=ORIENTED_EDGE('',*,*,#15544,.T.);
#21261=ORIENTED_EDGE('',*,*,#15544,.F.);
#21262=ORIENTED_EDGE('',*,*,#15545,.T.);
#21263=ORIENTED_EDGE('',*,*,#15538,.T.);
#21264=ORIENTED_EDGE('',*,*,#15545,.F.);
#21265=ORIENTED_EDGE('',*,*,#15486,.F.);
#21266=ORIENTED_EDGE('',*,*,#15546,.T.);
#21267=ORIENTED_EDGE('',*,*,#15504,.F.);
#21268=ORIENTED_EDGE('',*,*,#15546,.F.);
#21269=ORIENTED_EDGE('',*,*,#15459,.F.);
#21270=ORIENTED_EDGE('',*,*,#15547,.T.);
#21271=ORIENTED_EDGE('',*,*,#15474,.F.);
#21272=ORIENTED_EDGE('',*,*,#15548,.T.);
#21273=ORIENTED_EDGE('',*,*,#15456,.F.);
#21274=ORIENTED_EDGE('',*,*,#15548,.F.);
#21275=ORIENTED_EDGE('',*,*,#15477,.F.);
#21276=ORIENTED_EDGE('',*,*,#15549,.F.);
#21277=ORIENTED_EDGE('',*,*,#15453,.F.);
#21278=ORIENTED_EDGE('',*,*,#15549,.T.);
#21279=ORIENTED_EDGE('',*,*,#15480,.F.);
#21280=ORIENTED_EDGE('',*,*,#15550,.T.);
#21281=ORIENTED_EDGE('',*,*,#15448,.F.);
#21282=ORIENTED_EDGE('',*,*,#15551,.F.);
#21283=ORIENTED_EDGE('',*,*,#15552,.F.);
#21284=ORIENTED_EDGE('',*,*,#15467,.F.);
#21285=ORIENTED_EDGE('',*,*,#15451,.F.);
#21286=ORIENTED_EDGE('',*,*,#15550,.F.);
#21287=ORIENTED_EDGE('',*,*,#15483,.F.);
#21288=ORIENTED_EDGE('',*,*,#15553,.F.);
#21289=ORIENTED_EDGE('',*,*,#15551,.T.);
#21290=ORIENTED_EDGE('',*,*,#15462,.F.);
#21291=ORIENTED_EDGE('',*,*,#15466,.T.);
#21292=ORIENTED_EDGE('',*,*,#15554,.F.);
#21293=ORIENTED_EDGE('',*,*,#15472,.F.);
#21294=ORIENTED_EDGE('',*,*,#15547,.F.);
#21295=ORIENTED_EDGE('',*,*,#15468,.T.);
#21296=ORIENTED_EDGE('',*,*,#15555,.F.);
#21297=ORIENTED_EDGE('',*,*,#15505,.F.);
#21298=ORIENTED_EDGE('',*,*,#15522,.F.);
#21299=ORIENTED_EDGE('',*,*,#15556,.F.);
#21300=ORIENTED_EDGE('',*,*,#15557,.F.);
#21301=ORIENTED_EDGE('',*,*,#15506,.F.);
#21302=ORIENTED_EDGE('',*,*,#15557,.T.);
#21303=ORIENTED_EDGE('',*,*,#15558,.F.);
#21304=ORIENTED_EDGE('',*,*,#15529,.T.);
#21305=ORIENTED_EDGE('',*,*,#15520,.F.);
#21306=ORIENTED_EDGE('',*,*,#15517,.F.);
#21307=ORIENTED_EDGE('',*,*,#15514,.F.);
#21308=ORIENTED_EDGE('',*,*,#15511,.F.);
#21309=ORIENTED_EDGE('',*,*,#15558,.T.);
#21310=ORIENTED_EDGE('',*,*,#15559,.F.);
#21311=ORIENTED_EDGE('',*,*,#15554,.T.);
#21312=ORIENTED_EDGE('',*,*,#15560,.F.);
#21313=ORIENTED_EDGE('',*,*,#15561,.F.);
#21314=ORIENTED_EDGE('',*,*,#15521,.T.);
#21315=ORIENTED_EDGE('',*,*,#15500,.F.);
#21316=ORIENTED_EDGE('',*,*,#15503,.T.);
#21317=ORIENTED_EDGE('',*,*,#15487,.F.);
#21318=ORIENTED_EDGE('',*,*,#15528,.T.);
#21319=ORIENTED_EDGE('',*,*,#15562,.F.);
#21320=ORIENTED_EDGE('',*,*,#15553,.T.);
#21321=ORIENTED_EDGE('',*,*,#15482,.F.);
#21322=ORIENTED_EDGE('',*,*,#15485,.T.);
#21323=ORIENTED_EDGE('',*,*,#15469,.F.);
#21324=ORIENTED_EDGE('',*,*,#15561,.T.);
#21325=ORIENTED_EDGE('',*,*,#15563,.T.);
#21326=ORIENTED_EDGE('',*,*,#15564,.T.);
#21327=ORIENTED_EDGE('',*,*,#15563,.F.);
#21328=ORIENTED_EDGE('',*,*,#15560,.T.);
#21329=ORIENTED_EDGE('',*,*,#15465,.T.);
#21330=ORIENTED_EDGE('',*,*,#15555,.T.);
#21331=ORIENTED_EDGE('',*,*,#15552,.T.);
#21332=ORIENTED_EDGE('',*,*,#15562,.T.);
#21333=ORIENTED_EDGE('',*,*,#15530,.T.);
#21334=ORIENTED_EDGE('',*,*,#15559,.T.);
#21335=ORIENTED_EDGE('',*,*,#15556,.T.);
#21336=ORIENTED_EDGE('',*,*,#15564,.F.);
#21337=ORIENTED_EDGE('',*,*,#15565,.T.);
#21338=ORIENTED_EDGE('',*,*,#15404,.F.);
#21339=ORIENTED_EDGE('',*,*,#15565,.F.);
#21340=ORIENTED_EDGE('',*,*,#15566,.T.);
#21341=ORIENTED_EDGE('',*,*,#15567,.T.);
#21342=ORIENTED_EDGE('',*,*,#15568,.T.);
#21343=ORIENTED_EDGE('',*,*,#15567,.F.);
#21344=ORIENTED_EDGE('',*,*,#15569,.F.);
#21345=ORIENTED_EDGE('',*,*,#15570,.T.);
#21346=ORIENTED_EDGE('',*,*,#15568,.F.);
#21347=ORIENTED_EDGE('',*,*,#15570,.F.);
#21348=ORIENTED_EDGE('',*,*,#15571,.T.);
#21349=ORIENTED_EDGE('',*,*,#15566,.F.);
#21350=ORIENTED_EDGE('',*,*,#15572,.F.);
#21351=ORIENTED_EDGE('',*,*,#15414,.F.);
#21352=ORIENTED_EDGE('',*,*,#15410,.F.);
#21353=ORIENTED_EDGE('',*,*,#15406,.F.);
#21354=ORIENTED_EDGE('',*,*,#15573,.F.);
#21355=ORIENTED_EDGE('',*,*,#15408,.F.);
#21356=ORIENTED_EDGE('',*,*,#15412,.T.);
#21357=ORIENTED_EDGE('',*,*,#15413,.F.);
#21358=ORIENTED_EDGE('',*,*,#15569,.T.);
#21359=ORIENTED_EDGE('',*,*,#15574,.T.);
#21360=ORIENTED_EDGE('',*,*,#15575,.T.);
#21361=ORIENTED_EDGE('',*,*,#15403,.T.);
#21362=ORIENTED_EDGE('',*,*,#15575,.F.);
#21363=ORIENTED_EDGE('',*,*,#15576,.T.);
#21364=ORIENTED_EDGE('',*,*,#15577,.F.);
#21365=ORIENTED_EDGE('',*,*,#15578,.T.);
#21366=ORIENTED_EDGE('',*,*,#15576,.F.);
#21367=ORIENTED_EDGE('',*,*,#15574,.F.);
#21368=ORIENTED_EDGE('',*,*,#15578,.F.);
#21369=ORIENTED_EDGE('',*,*,#15573,.T.);
#21370=ORIENTED_EDGE('',*,*,#15415,.F.);
#21371=ORIENTED_EDGE('',*,*,#15572,.T.);
#21372=ORIENTED_EDGE('',*,*,#15409,.F.);
#21373=ORIENTED_EDGE('',*,*,#15579,.F.);
#21374=ORIENTED_EDGE('',*,*,#15577,.T.);
#21375=ORIENTED_EDGE('',*,*,#15580,.F.);
#21376=ORIENTED_EDGE('',*,*,#15581,.T.);
#21377=ORIENTED_EDGE('',*,*,#15579,.T.);
#21378=ORIENTED_EDGE('',*,*,#15581,.F.);
#21379=ORIENTED_EDGE('',*,*,#15582,.F.);
#21380=ORIENTED_EDGE('',*,*,#15583,.T.);
#21381=ORIENTED_EDGE('',*,*,#15580,.T.);
#21382=ORIENTED_EDGE('',*,*,#15583,.F.);
#21383=ORIENTED_EDGE('',*,*,#15571,.F.);
#21384=ORIENTED_EDGE('',*,*,#15584,.T.);
#21385=ORIENTED_EDGE('',*,*,#15582,.T.);
#21386=ORIENTED_EDGE('',*,*,#15584,.F.);
#21387=ORIENTED_EDGE('',*,*,#15585,.T.);
#21388=ORIENTED_EDGE('',*,*,#15440,.T.);
#21389=ORIENTED_EDGE('',*,*,#15586,.T.);
#21390=ORIENTED_EDGE('',*,*,#15587,.T.);
#21391=ORIENTED_EDGE('',*,*,#15588,.T.);
#21392=ORIENTED_EDGE('',*,*,#15437,.T.);
#21393=ORIENTED_EDGE('',*,*,#15585,.F.);
#21394=ORIENTED_EDGE('',*,*,#15589,.T.);
#21395=ORIENTED_EDGE('',*,*,#15590,.T.);
#21396=ORIENTED_EDGE('',*,*,#15591,.T.);
#21397=ORIENTED_EDGE('',*,*,#15588,.F.);
#21398=ORIENTED_EDGE('',*,*,#15592,.T.);
#21399=ORIENTED_EDGE('',*,*,#15593,.T.);
#21400=ORIENTED_EDGE('',*,*,#15594,.T.);
#21401=ORIENTED_EDGE('',*,*,#15590,.F.);
#21402=ORIENTED_EDGE('',*,*,#15595,.T.);
#21403=ORIENTED_EDGE('',*,*,#15596,.T.);
#21404=ORIENTED_EDGE('',*,*,#15597,.T.);
#21405=ORIENTED_EDGE('',*,*,#15593,.F.);
#21406=ORIENTED_EDGE('',*,*,#15598,.T.);
#21407=ORIENTED_EDGE('',*,*,#15599,.T.);
#21408=ORIENTED_EDGE('',*,*,#15600,.T.);
#21409=ORIENTED_EDGE('',*,*,#15596,.F.);
#21410=ORIENTED_EDGE('',*,*,#15601,.T.);
#21411=ORIENTED_EDGE('',*,*,#15602,.T.);
#21412=ORIENTED_EDGE('',*,*,#15444,.T.);
#21413=ORIENTED_EDGE('',*,*,#15599,.F.);
#21414=ORIENTED_EDGE('',*,*,#15603,.T.);
#21415=ORIENTED_EDGE('',*,*,#15586,.F.);
#21416=ORIENTED_EDGE('',*,*,#15442,.T.);
#21417=ORIENTED_EDGE('',*,*,#15602,.F.);
#21418=ORIENTED_EDGE('',*,*,#15604,.T.);
#21419=ORIENTED_EDGE('',*,*,#15435,.F.);
#21420=ORIENTED_EDGE('',*,*,#15605,.T.);
#21421=ORIENTED_EDGE('',*,*,#15600,.F.);
#21422=ORIENTED_EDGE('',*,*,#15443,.T.);
#21423=ORIENTED_EDGE('',*,*,#15587,.F.);
#21424=ORIENTED_EDGE('',*,*,#15604,.F.);
#21425=ORIENTED_EDGE('',*,*,#15603,.F.);
#21426=ORIENTED_EDGE('',*,*,#15601,.F.);
#21427=ORIENTED_EDGE('',*,*,#15598,.F.);
#21428=ORIENTED_EDGE('',*,*,#15595,.F.);
#21429=ORIENTED_EDGE('',*,*,#15592,.F.);
#21430=ORIENTED_EDGE('',*,*,#15589,.F.);
#21431=ORIENTED_EDGE('',*,*,#15381,.F.);
#21432=ORIENTED_EDGE('',*,*,#15606,.T.);
#21433=ORIENTED_EDGE('',*,*,#15427,.F.);
#21434=ORIENTED_EDGE('',*,*,#15446,.F.);
#21435=ORIENTED_EDGE('',*,*,#15384,.F.);
#21436=ORIENTED_EDGE('',*,*,#15396,.T.);
#21437=ORIENTED_EDGE('',*,*,#15424,.F.);
#21438=ORIENTED_EDGE('',*,*,#15606,.F.);
#21439=ORIENTED_EDGE('',*,*,#15434,.F.);
#21440=ORIENTED_EDGE('',*,*,#15607,.F.);
#21441=ORIENTED_EDGE('',*,*,#15597,.F.);
#21442=ORIENTED_EDGE('',*,*,#15605,.F.);
#21443=ORIENTED_EDGE('',*,*,#15431,.F.);
#21444=ORIENTED_EDGE('',*,*,#15608,.T.);
#21445=ORIENTED_EDGE('',*,*,#15594,.F.);
#21446=ORIENTED_EDGE('',*,*,#15607,.T.);
#21447=ORIENTED_EDGE('',*,*,#15428,.F.);
#21448=ORIENTED_EDGE('',*,*,#15438,.F.);
#21449=ORIENTED_EDGE('',*,*,#15591,.F.);
#21450=ORIENTED_EDGE('',*,*,#15608,.F.);
#26400=PLANE('',#29350);
#26401=PLANE('',#29354);
#26402=PLANE('',#29358);
#26403=PLANE('',#29362);
#26404=PLANE('',#29363);
#26405=PLANE('',#29366);
#26406=PLANE('',#29369);
#26407=PLANE('',#29373);
#26408=PLANE('',#29377);
#26409=PLANE('',#29378);
#26410=PLANE('',#29381);
#26411=PLANE('',#29385);
#26412=PLANE('',#29389);
#26413=PLANE('',#29394);
#26414=PLANE('',#29397);
#26415=PLANE('',#29400);
#26416=PLANE('',#29401);
#26417=PLANE('',#29405);
#26418=PLANE('',#29409);
#26419=PLANE('',#29410);
#26420=PLANE('',#29412);
#26421=PLANE('',#29413);
#26422=PLANE('',#29417);
#26423=PLANE('',#29421);
#26424=PLANE('',#29422);
#26425=PLANE('',#29424);
#26426=PLANE('',#29428);
#26427=PLANE('',#29432);
#26428=PLANE('',#29433);
#26429=PLANE('',#29435);
#26430=PLANE('',#29439);
#26431=PLANE('',#29443);
#26432=PLANE('',#29444);
#26433=PLANE('',#29446);
#26434=PLANE('',#29448);
#26435=PLANE('',#29449);
#26436=PLANE('',#29454);
#26437=PLANE('',#29469);
#26438=PLANE('',#29471);
#26439=PLANE('',#29473);
#26440=PLANE('',#29474);
#26441=PLANE('',#29475);
#26442=PLANE('',#29477);
#26443=PLANE('',#29479);
#26444=PLANE('',#29480);
#26445=PLANE('',#29482);
#26446=PLANE('',#29494);
#26447=PLANE('',#29496);
#26448=PLANE('',#29498);
#26449=PLANE('',#29500);
#26450=PLANE('',#29507);
#26451=PLANE('',#29514);
#26452=PLANE('',#29517);
#26453=PLANE('',#29521);
#26454=PLANE('',#29525);
#26455=PLANE('',#29529);
#26456=PLANE('',#29530);
#26457=PLANE('',#29532);
#26458=PLANE('',#29534);
#27445=ADVANCED_FACE('',(#3537),#2819,.T.);
#27446=ADVANCED_FACE('',(#3538),#26400,.T.);
#27447=ADVANCED_FACE('',(#3539),#2820,.T.);
#27448=ADVANCED_FACE('',(#3540),#26401,.T.);
#27449=ADVANCED_FACE('',(#3541),#2821,.T.);
#27450=ADVANCED_FACE('',(#3542),#26402,.T.);
#27451=ADVANCED_FACE('',(#3543),#2822,.T.);
#27452=ADVANCED_FACE('',(#3544),#26403,.T.);
#27453=ADVANCED_FACE('',(#3545),#26404,.T.);
#27454=ADVANCED_FACE('',(#3546),#2823,.T.);
#27455=ADVANCED_FACE('',(#3547),#26405,.T.);
#27456=ADVANCED_FACE('',(#3548),#2824,.T.);
#27457=ADVANCED_FACE('',(#3549,#1918,#1919,#1920),#26406,.T.);
#27458=ADVANCED_FACE('',(#3550),#26407,.T.);
#27459=ADVANCED_FACE('',(#3551),#1575,.F.);
#27460=ADVANCED_FACE('',(#3552),#26408,.T.);
#27461=ADVANCED_FACE('',(#3553),#26409,.T.);
#27462=ADVANCED_FACE('',(#3554),#2825,.T.);
#27463=ADVANCED_FACE('',(#3555),#26410,.T.);
#27464=ADVANCED_FACE('',(#3556),#2826,.T.);
#27465=ADVANCED_FACE('',(#3557),#26411,.T.);
#27466=ADVANCED_FACE('',(#3558),#2827,.T.);
#27467=ADVANCED_FACE('',(#3559),#26412,.T.);
#27468=ADVANCED_FACE('',(#3560),#2828,.T.);
#27469=ADVANCED_FACE('',(#3561),#1576,.T.);
#27470=ADVANCED_FACE('',(#3562),#26413,.T.);
#27471=ADVANCED_FACE('',(#3563),#1577,.T.);
#27472=ADVANCED_FACE('',(#3564,#1921),#26414,.T.);
#27473=ADVANCED_FACE('',(#3565),#2829,.T.);
#27474=ADVANCED_FACE('',(#3566),#26415,.T.);
#27475=ADVANCED_FACE('',(#3567),#26416,.T.);
#27476=ADVANCED_FACE('',(#3568),#2830,.T.);
#27477=ADVANCED_FACE('',(#3569),#26417,.T.);
#27478=ADVANCED_FACE('',(#3570),#2831,.T.);
#27479=ADVANCED_FACE('',(#3571),#26418,.T.);
#27480=ADVANCED_FACE('',(#3572),#26419,.F.);
#27481=ADVANCED_FACE('',(#3573),#26420,.T.);
#27482=ADVANCED_FACE('',(#3574),#26421,.T.);
#27483=ADVANCED_FACE('',(#3575),#2832,.T.);
#27484=ADVANCED_FACE('',(#3576),#26422,.T.);
#27485=ADVANCED_FACE('',(#3577),#2833,.T.);
#27486=ADVANCED_FACE('',(#3578),#26423,.T.);
#27487=ADVANCED_FACE('',(#3579,#1922),#26424,.T.);
#27488=ADVANCED_FACE('',(#3580),#26425,.T.);
#27489=ADVANCED_FACE('',(#3581),#2834,.T.);
#27490=ADVANCED_FACE('',(#3582),#26426,.T.);
#27491=ADVANCED_FACE('',(#3583),#2835,.T.);
#27492=ADVANCED_FACE('',(#3584),#26427,.T.);
#27493=ADVANCED_FACE('',(#3585,#1923),#26428,.T.);
#27494=ADVANCED_FACE('',(#3586),#26429,.T.);
#27495=ADVANCED_FACE('',(#3587),#2836,.T.);
#27496=ADVANCED_FACE('',(#3588),#26430,.T.);
#27497=ADVANCED_FACE('',(#3589),#2837,.T.);
#27498=ADVANCED_FACE('',(#3590),#26431,.T.);
#27499=ADVANCED_FACE('',(#3591),#26432,.T.);
#27500=ADVANCED_FACE('',(#3592),#1578,.T.);
#27501=ADVANCED_FACE('',(#3593),#26433,.T.);
#27502=ADVANCED_FACE('',(#3594),#1579,.T.);
#27503=ADVANCED_FACE('',(#3595),#26434,.T.);
#27504=ADVANCED_FACE('',(#3596),#26435,.F.);
#27505=ADVANCED_FACE('',(#3597),#2838,.T.);
#27506=ADVANCED_FACE('',(#3598,#1924),#26436,.T.);
#27507=ADVANCED_FACE('',(#3599),#1580,.T.);
#27508=ADVANCED_FACE('',(#3600),#2839,.F.);
#27509=ADVANCED_FACE('',(#3601),#1581,.F.);
#27510=ADVANCED_FACE('',(#3602),#2840,.F.);
#27511=ADVANCED_FACE('',(#3603),#1582,.F.);
#27512=ADVANCED_FACE('',(#3604),#2841,.F.);
#27513=ADVANCED_FACE('',(#3605),#2842,.F.);
#27514=ADVANCED_FACE('',(#3606),#1583,.T.);
#27515=ADVANCED_FACE('',(#3607),#1584,.T.);
#27516=ADVANCED_FACE('',(#3608),#26437,.T.);
#27517=ADVANCED_FACE('',(#3609),#1585,.T.);
#27518=ADVANCED_FACE('',(#3610),#26438,.F.);
#27519=ADVANCED_FACE('',(#3611),#26439,.T.);
#27520=ADVANCED_FACE('',(#3612),#26440,.T.);
#27521=ADVANCED_FACE('',(#3613),#26441,.T.);
#27522=ADVANCED_FACE('',(#3614),#26442,.F.);
#27523=ADVANCED_FACE('',(#3615),#26443,.T.);
#27524=ADVANCED_FACE('',(#3616),#26444,.T.);
#27525=ADVANCED_FACE('',(#3617),#26445,.T.);
#27526=ADVANCED_FACE('',(#3618),#2843,.T.);
#27527=ADVANCED_FACE('',(#3619),#1586,.T.);
#27528=ADVANCED_FACE('',(#3620),#2844,.F.);
#27529=ADVANCED_FACE('',(#3621),#1587,.F.);
#27530=ADVANCED_FACE('',(#3622,#1925),#26446,.T.);
#27531=ADVANCED_FACE('',(#3623),#26447,.F.);
#27532=ADVANCED_FACE('',(#3624),#26448,.F.);
#27533=ADVANCED_FACE('',(#3625),#26449,.F.);
#27534=ADVANCED_FACE('',(#3626),#376,.F.);
#27535=ADVANCED_FACE('',(#3627,#1926),#1588,.T.);
#27536=ADVANCED_FACE('',(#3628,#1927),#26450,.T.);
#27537=ADVANCED_FACE('',(#3629),#2845,.T.);
#27538=ADVANCED_FACE('',(#3630),#1589,.T.);
#27539=ADVANCED_FACE('',(#3631),#2846,.T.);
#27540=ADVANCED_FACE('',(#3632),#26451,.T.);
#27541=ADVANCED_FACE('',(#3633),#2847,.T.);
#27542=ADVANCED_FACE('',(#3634),#26452,.T.);
#27543=ADVANCED_FACE('',(#3635),#2848,.T.);
#27544=ADVANCED_FACE('',(#3636),#26453,.T.);
#27545=ADVANCED_FACE('',(#3637),#2849,.T.);
#27546=ADVANCED_FACE('',(#3638),#26454,.T.);
#27547=ADVANCED_FACE('',(#3639),#2850,.T.);
#27548=ADVANCED_FACE('',(#3640),#1590,.T.);
#27549=ADVANCED_FACE('',(#3641),#26455,.F.);
#27550=ADVANCED_FACE('',(#3642),#26456,.T.);
#27551=ADVANCED_FACE('',(#3643),#2851,.T.);
#27552=ADVANCED_FACE('',(#3644),#26457,.T.);
#27553=ADVANCED_FACE('',(#3645),#1591,.T.);
#27554=ADVANCED_FACE('',(#3646),#26458,.T.);
#28463=CLOSED_SHELL('',(#27445,#27446,#27447,#27448,#27449,#27450,#27451,
#27452,#27453,#27454,#27455,#27456,#27457,#27458,#27459,#27460,#27461,#27462,
#27463,#27464,#27465,#27466,#27467,#27468,#27469,#27470,#27471,#27472,#27473,
#27474,#27475,#27476,#27477,#27478,#27479,#27480,#27481,#27482,#27483,#27484,
#27485,#27486,#27487,#27488,#27489,#27490,#27491,#27492,#27493,#27494,#27495,
#27496,#27497,#27498,#27499,#27500,#27501,#27502,#27503,#27504,#27505,#27506,
#27507,#27508,#27509,#27510,#27511,#27512,#27513,#27514,#27515,#27516,#27517,
#27518,#27519,#27520,#27521,#27522,#27523,#27524,#27525,#27526,#27527,#27528,
#27529,#27530,#27531,#27532,#27533,#27534,#27535,#27536,#27537,#27538,#27539,
#27540,#27541,#27542,#27543,#27544,#27545,#27546,#27547,#27548,#27549,#27550,
#27551,#27552,#27553,#27554));
#29346=AXIS2_PLACEMENT_3D('',#43529,#33271,#33272);
#29347=AXIS2_PLACEMENT_3D('',#43530,#33273,#33274);
#29348=AXIS2_PLACEMENT_3D('',#43535,#33276,#33277);
#29349=AXIS2_PLACEMENT_3D('',#43538,#33279,#33280);
#29350=AXIS2_PLACEMENT_3D('',#43539,#33281,#33282);
#29351=AXIS2_PLACEMENT_3D('',#43545,#33286,#33287);
#29352=AXIS2_PLACEMENT_3D('',#43549,#33289,#33290);
#29353=AXIS2_PLACEMENT_3D('',#43550,#33291,#33292);
#29354=AXIS2_PLACEMENT_3D('',#43551,#33293,#33294);
#29355=AXIS2_PLACEMENT_3D('',#43557,#33298,#33299);
#29356=AXIS2_PLACEMENT_3D('',#43561,#33301,#33302);
#29357=AXIS2_PLACEMENT_3D('',#43562,#33303,#33304);
#29358=AXIS2_PLACEMENT_3D('',#43563,#33305,#33306);
#29359=AXIS2_PLACEMENT_3D('',#43569,#33310,#33311);
#29360=AXIS2_PLACEMENT_3D('',#43573,#33313,#33314);
#29361=AXIS2_PLACEMENT_3D('',#43574,#33315,#33316);
#29362=AXIS2_PLACEMENT_3D('',#43575,#33317,#33318);
#29363=AXIS2_PLACEMENT_3D('',#43578,#33321,#33322);
#29364=AXIS2_PLACEMENT_3D('',#43584,#33326,#33327);
#29365=AXIS2_PLACEMENT_3D('',#43587,#33329,#33330);
#29366=AXIS2_PLACEMENT_3D('',#43588,#33331,#33332);
#29367=AXIS2_PLACEMENT_3D('',#43592,#33335,#33336);
#29368=AXIS2_PLACEMENT_3D('',#43595,#33338,#33339);
#29369=AXIS2_PLACEMENT_3D('',#43596,#33340,#33341);
#29370=AXIS2_PLACEMENT_3D('',#43598,#33342,#33343);
#29371=AXIS2_PLACEMENT_3D('',#43600,#33344,#33345);
#29372=AXIS2_PLACEMENT_3D('',#43602,#33346,#33347);
#29373=AXIS2_PLACEMENT_3D('',#43603,#33348,#33349);
#29374=AXIS2_PLACEMENT_3D('',#43612,#33354,#33355);
#29375=AXIS2_PLACEMENT_3D('',#43614,#33356,#33357);
#29376=AXIS2_PLACEMENT_3D('',#43617,#33359,#33360);
#29377=AXIS2_PLACEMENT_3D('',#43618,#33361,#33362);
#29378=AXIS2_PLACEMENT_3D('',#43624,#33366,#33367);
#29379=AXIS2_PLACEMENT_3D('',#43630,#33371,#33372);
#29380=AXIS2_PLACEMENT_3D('',#43633,#33374,#33375);
#29381=AXIS2_PLACEMENT_3D('',#43634,#33376,#33377);
#29382=AXIS2_PLACEMENT_3D('',#43638,#33380,#33381);
#29383=AXIS2_PLACEMENT_3D('',#43642,#33383,#33384);
#29384=AXIS2_PLACEMENT_3D('',#43643,#33385,#33386);
#29385=AXIS2_PLACEMENT_3D('',#43644,#33387,#33388);
#29386=AXIS2_PLACEMENT_3D('',#43650,#33392,#33393);
#29387=AXIS2_PLACEMENT_3D('',#43654,#33395,#33396);
#29388=AXIS2_PLACEMENT_3D('',#43655,#33397,#33398);
#29389=AXIS2_PLACEMENT_3D('',#43656,#33399,#33400);
#29390=AXIS2_PLACEMENT_3D('',#43661,#33404,#33405);
#29391=AXIS2_PLACEMENT_3D('',#43662,#33406,#33407);
#29392=AXIS2_PLACEMENT_3D('',#43663,#33408,#33409);
#29393=AXIS2_PLACEMENT_3D('',#43667,#33411,#33412);
#29394=AXIS2_PLACEMENT_3D('',#43669,#33414,#33415);
#29395=AXIS2_PLACEMENT_3D('',#43673,#33418,#33419);
#29396=AXIS2_PLACEMENT_3D('',#43676,#33421,#33422);
#29397=AXIS2_PLACEMENT_3D('',#43677,#33423,#33424);
#29398=AXIS2_PLACEMENT_3D('',#43682,#33427,#33428);
#29399=AXIS2_PLACEMENT_3D('',#43683,#33429,#33430);
#29400=AXIS2_PLACEMENT_3D('',#43686,#33433,#33434);
#29401=AXIS2_PLACEMENT_3D('',#43687,#33435,#33436);
#29402=AXIS2_PLACEMENT_3D('',#43696,#33441,#33442);
#29403=AXIS2_PLACEMENT_3D('',#43700,#33444,#33445);
#29404=AXIS2_PLACEMENT_3D('',#43701,#33446,#33447);
#29405=AXIS2_PLACEMENT_3D('',#43702,#33448,#33449);
#29406=AXIS2_PLACEMENT_3D('',#43708,#33453,#33454);
#29407=AXIS2_PLACEMENT_3D('',#43712,#33456,#33457);
#29408=AXIS2_PLACEMENT_3D('',#43713,#33458,#33459);
#29409=AXIS2_PLACEMENT_3D('',#43714,#33460,#33461);
#29410=AXIS2_PLACEMENT_3D('',#43720,#33465,#33466);
#29411=AXIS2_PLACEMENT_3D('',#43724,#33468,#33469);
#29412=AXIS2_PLACEMENT_3D('',#43726,#33471,#33472);
#29413=AXIS2_PLACEMENT_3D('',#43730,#33475,#33476);
#29414=AXIS2_PLACEMENT_3D('',#43739,#33481,#33482);
#29415=AXIS2_PLACEMENT_3D('',#43743,#33484,#33485);
#29416=AXIS2_PLACEMENT_3D('',#43744,#33486,#33487);
#29417=AXIS2_PLACEMENT_3D('',#43745,#33488,#33489);
#29418=AXIS2_PLACEMENT_3D('',#43751,#33493,#33494);
#29419=AXIS2_PLACEMENT_3D('',#43755,#33496,#33497);
#29420=AXIS2_PLACEMENT_3D('',#43756,#33498,#33499);
#29421=AXIS2_PLACEMENT_3D('',#43757,#33500,#33501);
#29422=AXIS2_PLACEMENT_3D('',#43763,#33505,#33506);
#29423=AXIS2_PLACEMENT_3D('',#43766,#33508,#33509);
#29424=AXIS2_PLACEMENT_3D('',#43767,#33510,#33511);
#29425=AXIS2_PLACEMENT_3D('',#43776,#33516,#33517);
#29426=AXIS2_PLACEMENT_3D('',#43780,#33519,#33520);
#29427=AXIS2_PLACEMENT_3D('',#43781,#33521,#33522);
#29428=AXIS2_PLACEMENT_3D('',#43782,#33523,#33524);
#29429=AXIS2_PLACEMENT_3D('',#43788,#33528,#33529);
#29430=AXIS2_PLACEMENT_3D('',#43792,#33531,#33532);
#29431=AXIS2_PLACEMENT_3D('',#43793,#33533,#33534);
#29432=AXIS2_PLACEMENT_3D('',#43794,#33535,#33536);
#29433=AXIS2_PLACEMENT_3D('',#43800,#33540,#33541);
#29434=AXIS2_PLACEMENT_3D('',#43803,#33543,#33544);
#29435=AXIS2_PLACEMENT_3D('',#43804,#33545,#33546);
#29436=AXIS2_PLACEMENT_3D('',#43813,#33551,#33552);
#29437=AXIS2_PLACEMENT_3D('',#43817,#33554,#33555);
#29438=AXIS2_PLACEMENT_3D('',#43818,#33556,#33557);
#29439=AXIS2_PLACEMENT_3D('',#43819,#33558,#33559);
#29440=AXIS2_PLACEMENT_3D('',#43825,#33563,#33564);
#29441=AXIS2_PLACEMENT_3D('',#43829,#33566,#33567);
#29442=AXIS2_PLACEMENT_3D('',#43830,#33568,#33569);
#29443=AXIS2_PLACEMENT_3D('',#43831,#33570,#33571);
#29444=AXIS2_PLACEMENT_3D('',#43837,#33575,#33576);
#29445=AXIS2_PLACEMENT_3D('',#43842,#33580,#33581);
#29446=AXIS2_PLACEMENT_3D('',#43844,#33583,#33584);
#29447=AXIS2_PLACEMENT_3D('',#43846,#33586,#33587);
#29448=AXIS2_PLACEMENT_3D('',#43848,#33589,#33590);
#29449=AXIS2_PLACEMENT_3D('',#43852,#33593,#33594);
#29450=AXIS2_PLACEMENT_3D('',#43855,#33596,#33597);
#29451=AXIS2_PLACEMENT_3D('',#43856,#33598,#33599);
#29452=AXIS2_PLACEMENT_3D('',#43858,#33600,#33601);
#29453=AXIS2_PLACEMENT_3D('',#43861,#33603,#33604);
#29454=AXIS2_PLACEMENT_3D('',#43862,#33605,#33606);
#29455=AXIS2_PLACEMENT_3D('',#43864,#33607,#33608);
#29456=AXIS2_PLACEMENT_3D('',#43865,#33609,#33610);
#29457=AXIS2_PLACEMENT_3D('',#43867,#33612,#33613);
#29458=AXIS2_PLACEMENT_3D('',#43870,#33615,#33616);
#29459=AXIS2_PLACEMENT_3D('',#43871,#33617,#33618);
#29460=AXIS2_PLACEMENT_3D('',#43873,#33619,#33620);
#29461=AXIS2_PLACEMENT_3D('',#43875,#33622,#33623);
#29462=AXIS2_PLACEMENT_3D('',#43878,#33625,#33626);
#29463=AXIS2_PLACEMENT_3D('',#43879,#33627,#33628);
#29464=AXIS2_PLACEMENT_3D('',#43882,#33630,#33631);
#29465=AXIS2_PLACEMENT_3D('',#43883,#33632,#33633);
#29466=AXIS2_PLACEMENT_3D('',#43886,#33635,#33636);
#29467=AXIS2_PLACEMENT_3D('',#43889,#33638,#33639);
#29468=AXIS2_PLACEMENT_3D('',#43891,#33641,#33642);
#29469=AXIS2_PLACEMENT_3D('',#43894,#33645,#33646);
#29470=AXIS2_PLACEMENT_3D('',#43896,#33648,#33649);
#29471=AXIS2_PLACEMENT_3D('',#43898,#33651,#33652);
#29472=AXIS2_PLACEMENT_3D('',#43901,#33654,#33655);
#29473=AXIS2_PLACEMENT_3D('',#43902,#33656,#33657);
#29474=AXIS2_PLACEMENT_3D('',#43904,#33659,#33660);
#29475=AXIS2_PLACEMENT_3D('',#43906,#33662,#33663);
#29476=AXIS2_PLACEMENT_3D('',#43907,#33664,#33665);
#29477=AXIS2_PLACEMENT_3D('',#43908,#33666,#33667);
#29478=AXIS2_PLACEMENT_3D('',#43910,#33668,#33669);
#29479=AXIS2_PLACEMENT_3D('',#43912,#33671,#33672);
#29480=AXIS2_PLACEMENT_3D('',#43914,#33674,#33675);
#29481=AXIS2_PLACEMENT_3D('',#43915,#33676,#33677);
#29482=AXIS2_PLACEMENT_3D('',#43916,#33678,#33679);
#29483=AXIS2_PLACEMENT_3D('',#43918,#33680,#33681);
#29484=AXIS2_PLACEMENT_3D('',#43919,#33682,#33683);
#29485=AXIS2_PLACEMENT_3D('',#43920,#33684,#33685);
#29486=AXIS2_PLACEMENT_3D('',#43921,#33686,#33687);
#29487=AXIS2_PLACEMENT_3D('',#43924,#33689,#33690);
#29488=AXIS2_PLACEMENT_3D('',#43925,#33691,#33692);
#29489=AXIS2_PLACEMENT_3D('',#43927,#33694,#33695);
#29490=AXIS2_PLACEMENT_3D('',#43929,#33696,#33697);
#29491=AXIS2_PLACEMENT_3D('',#43932,#33699,#33700);
#29492=AXIS2_PLACEMENT_3D('',#43933,#33701,#33702);
#29493=AXIS2_PLACEMENT_3D('',#43935,#33703,#33704);
#29494=AXIS2_PLACEMENT_3D('',#43937,#33706,#33707);
#29495=AXIS2_PLACEMENT_3D('',#43939,#33708,#33709);
#29496=AXIS2_PLACEMENT_3D('',#43940,#33710,#33711);
#29497=AXIS2_PLACEMENT_3D('',#43941,#33712,#33713);
#29498=AXIS2_PLACEMENT_3D('',#43942,#33714,#33715);
#29499=AXIS2_PLACEMENT_3D('',#43943,#33716,#33717);
#29500=AXIS2_PLACEMENT_3D('',#43944,#33718,#33719);
#29501=AXIS2_PLACEMENT_3D('',#43945,#33720,#33721);
#29502=AXIS2_PLACEMENT_3D('',#43948,#33722,#33723);
#29503=AXIS2_PLACEMENT_3D('',#43949,#33724,#33725);
#29504=AXIS2_PLACEMENT_3D('',#43950,#33726,#33727);
#29505=AXIS2_PLACEMENT_3D('',#43951,#33728,#33729);
#29506=AXIS2_PLACEMENT_3D('',#43953,#33730,#33731);
#29507=AXIS2_PLACEMENT_3D('',#43955,#33733,#33734);
#29508=AXIS2_PLACEMENT_3D('',#43957,#33735,#33736);
#29509=AXIS2_PLACEMENT_3D('',#43958,#33737,#33738);
#29510=AXIS2_PLACEMENT_3D('',#43960,#33739,#33740);
#29511=AXIS2_PLACEMENT_3D('',#43962,#33742,#33743);
#29512=AXIS2_PLACEMENT_3D('',#43964,#33744,#33745);
#29513=AXIS2_PLACEMENT_3D('',#43966,#33747,#33748);
#29514=AXIS2_PLACEMENT_3D('',#43968,#33750,#33751);
#29515=AXIS2_PLACEMENT_3D('',#43974,#33755,#33756);
#29516=AXIS2_PLACEMENT_3D('',#43977,#33758,#33759);
#29517=AXIS2_PLACEMENT_3D('',#43978,#33760,#33761);
#29518=AXIS2_PLACEMENT_3D('',#43984,#33765,#33766);
#29519=AXIS2_PLACEMENT_3D('',#43988,#33768,#33769);
#29520=AXIS2_PLACEMENT_3D('',#43989,#33770,#33771);
#29521=AXIS2_PLACEMENT_3D('',#43990,#33772,#33773);
#29522=AXIS2_PLACEMENT_3D('',#43996,#33777,#33778);
#29523=AXIS2_PLACEMENT_3D('',#43999,#33780,#33781);
#29524=AXIS2_PLACEMENT_3D('',#44000,#33782,#33783);
#29525=AXIS2_PLACEMENT_3D('',#44001,#33784,#33785);
#29526=AXIS2_PLACEMENT_3D('',#44005,#33788,#33789);
#29527=AXIS2_PLACEMENT_3D('',#44006,#33790,#33791);
#29528=AXIS2_PLACEMENT_3D('',#44007,#33792,#33793);
#29529=AXIS2_PLACEMENT_3D('',#44009,#33795,#33796);
#29530=AXIS2_PLACEMENT_3D('',#44010,#33797,#33798);
#29531=AXIS2_PLACEMENT_3D('',#44012,#33800,#33801);
#29532=AXIS2_PLACEMENT_3D('',#44013,#33802,#33803);
#29533=AXIS2_PLACEMENT_3D('',#44015,#33805,#33806);
#29534=AXIS2_PLACEMENT_3D('',#44017,#33808,#33809);
#33271=DIRECTION('axis',(0.,0.,1.));
#33272=DIRECTION('refdir',(1.,0.,0.));
#33273=DIRECTION('center_axis',(0.,0.,-1.));
#33274=DIRECTION('ref_axis',(-0.707106781186547,-0.707106781186547,0.));
#33275=DIRECTION('',(-0.92387953251128,0.,-0.382683432365106));
#33276=DIRECTION('center_axis',(0.,0.,1.));
#33277=DIRECTION('ref_axis',(-0.707106781186547,-0.707106781186547,0.));
#33278=DIRECTION('',(0.,0.92387953251128,0.382683432365106));
#33279=DIRECTION('center_axis',(0.,0.,-1.));
#33280=DIRECTION('ref_axis',(-0.707106781186547,-0.707106781186547,0.));
#33281=DIRECTION('center_axis',(-0.382683432365179,0.,0.92387953251125));
#33282=DIRECTION('ref_axis',(0.92387953251125,0.,0.382683432365179));
#33283=DIRECTION('',(-0.923879532511251,0.,-0.382683432365176));
#33284=DIRECTION('',(0.,-1.,0.));
#33285=DIRECTION('',(0.,1.,0.));
#33286=DIRECTION('center_axis',(0.,0.,-1.));
#33287=DIRECTION('ref_axis',(-0.707106781186547,0.707106781186547,0.));
#33288=DIRECTION('',(0.,0.923879532511307,-0.382683432365041));
#33289=DIRECTION('center_axis',(0.,0.,1.));
#33290=DIRECTION('ref_axis',(-0.707106781186547,0.707106781186547,0.));
#33291=DIRECTION('center_axis',(0.,0.,-1.));
#33292=DIRECTION('ref_axis',(-0.707106781186547,0.707106781186547,0.));
#33293=DIRECTION('center_axis',(0.,0.382683432365181,0.923879532511249));
#33294=DIRECTION('ref_axis',(1.,0.,0.));
#33295=DIRECTION('',(0.,0.923879532511251,-0.382683432365176));
#33296=DIRECTION('',(-1.,0.,0.));
#33297=DIRECTION('',(1.,0.,0.));
#33298=DIRECTION('center_axis',(0.,0.,-1.));
#33299=DIRECTION('ref_axis',(0.707106781186547,0.707106781186547,0.));
#33300=DIRECTION('',(0.92387953251128,0.,-0.382683432365106));
#33301=DIRECTION('center_axis',(0.,0.,1.));
#33302=DIRECTION('ref_axis',(0.707106781186547,0.707106781186547,0.));
#33303=DIRECTION('center_axis',(0.,0.,-1.));
#33304=DIRECTION('ref_axis',(0.707106781186547,0.707106781186547,0.));
#33305=DIRECTION('center_axis',(0.382683432365179,0.,0.92387953251125));
#33306=DIRECTION('ref_axis',(0.92387953251125,0.,-0.382683432365179));
#33307=DIRECTION('',(0.923879532511251,0.,-0.382683432365176));
#33308=DIRECTION('',(0.,1.,0.));
#33309=DIRECTION('',(0.,-1.,0.));
#33310=DIRECTION('center_axis',(0.,0.,-1.));
#33311=DIRECTION('ref_axis',(0.707106781186547,-0.707106781186547,0.));
#33312=DIRECTION('',(0.,-0.92387953251128,-0.382683432365106));
#33313=DIRECTION('center_axis',(0.,0.,1.));
#33314=DIRECTION('ref_axis',(0.707106781186547,-0.707106781186547,0.));
#33315=DIRECTION('center_axis',(0.,0.,-1.));
#33316=DIRECTION('ref_axis',(0.707106781186547,-0.707106781186547,0.));
#33317=DIRECTION('center_axis',(0.,-0.382683432365179,0.92387953251125));
#33318=DIRECTION('ref_axis',(1.,0.,0.));
#33319=DIRECTION('',(1.,0.,0.));
#33320=DIRECTION('',(-1.,0.,0.));
#33321=DIRECTION('center_axis',(0.70710678118656,0.,0.707106781186535));
#33322=DIRECTION('ref_axis',(0.707106781186535,0.,-0.70710678118656));
#33323=DIRECTION('',(0.707106781186535,0.,-0.70710678118656));
#33324=DIRECTION('',(0.,-1.,0.));
#33325=DIRECTION('',(0.707106781186552,0.,-0.707106781186543));
#33326=DIRECTION('center_axis',(0.,0.,-1.));
#33327=DIRECTION('ref_axis',(0.707106781186548,-0.707106781186548,0.));
#33328=DIRECTION('',(0.,-0.707106781186552,-0.707106781186543));
#33329=DIRECTION('center_axis',(0.,0.,-1.));
#33330=DIRECTION('ref_axis',(0.707106781186548,-0.707106781186548,0.));
#33331=DIRECTION('center_axis',(0.,-0.70710678118656,0.707106781186535));
#33332=DIRECTION('ref_axis',(1.,0.,0.));
#33333=DIRECTION('',(0.,0.707106781186552,0.707106781186543));
#33334=DIRECTION('',(-1.,0.,0.));
#33335=DIRECTION('center_axis',(0.,0.,-1.));
#33336=DIRECTION('ref_axis',(-0.707106781186548,-0.707106781186548,0.));
#33337=DIRECTION('',(-0.707106781186552,0.,-0.707106781186543));
#33338=DIRECTION('center_axis',(0.,0.,-1.));
#33339=DIRECTION('ref_axis',(-0.707106781186548,-0.707106781186548,0.));
#33340=DIRECTION('center_axis',(0.,0.,1.));
#33341=DIRECTION('ref_axis',(1.,0.,0.));
#33342=DIRECTION('center_axis',(0.,0.,1.));
#33343=DIRECTION('ref_axis',(1.,0.,0.));
#33344=DIRECTION('center_axis',(0.,0.,-1.));
#33345=DIRECTION('ref_axis',(1.,0.,0.));
#33346=DIRECTION('center_axis',(0.,0.,-1.));
#33347=DIRECTION('ref_axis',(1.,0.,0.));
#33348=DIRECTION('center_axis',(0.490712016224176,-0.871321821793305,0.));
#33349=DIRECTION('ref_axis',(0.,0.,-1.));
#33350=DIRECTION('',(0.871321821793305,0.490712016224176,0.));
#33351=DIRECTION('',(0.,0.,-1.));
#33352=DIRECTION('',(-0.871321821793305,-0.490712016224176,0.));
#33353=DIRECTION('',(0.,0.,1.));
#33354=DIRECTION('center_axis',(0.,0.,1.));
#33355=DIRECTION('ref_axis',(-1.,1.22464679914735E-16,0.));
#33356=DIRECTION('center_axis',(0.,0.,1.));
#33357=DIRECTION('ref_axis',(1.,0.,0.));
#33358=DIRECTION('',(0.,0.,1.));
#33359=DIRECTION('center_axis',(0.,0.,1.));
#33360=DIRECTION('ref_axis',(1.,0.,0.));
#33361=DIRECTION('center_axis',(0.490712016224176,0.871321821793305,0.));
#33362=DIRECTION('ref_axis',(0.,0.,1.));
#33363=DIRECTION('',(0.871321821793305,-0.490712016224176,0.));
#33364=DIRECTION('',(-0.871321821793305,0.490712016224176,0.));
#33365=DIRECTION('',(0.,0.,-1.));
#33366=DIRECTION('center_axis',(0.,-0.923879532511285,0.382683432365094));
#33367=DIRECTION('ref_axis',(0.,-0.382683432365094,-0.923879532511285));
#33368=DIRECTION('',(0.,0.382683432365069,0.923879532511296));
#33369=DIRECTION('',(0.,-0.382683432365069,-0.923879532511296));
#33370=DIRECTION('',(1.,0.,0.));
#33371=DIRECTION('center_axis',(0.,0.,-1.));
#33372=DIRECTION('ref_axis',(0.707106781186548,-0.707106781186548,0.));
#33373=DIRECTION('',(-0.38268343236511,0.,0.923879532511279));
#33374=DIRECTION('center_axis',(0.,0.,1.));
#33375=DIRECTION('ref_axis',(0.707106781186548,-0.707106781186548,0.));
#33376=DIRECTION('center_axis',(0.923879532511285,0.,0.382683432365094));
#33377=DIRECTION('ref_axis',(0.382683432365094,0.,-0.923879532511285));
#33378=DIRECTION('',(-0.382683432365069,0.,0.923879532511296));
#33379=DIRECTION('',(0.,1.,0.));
#33380=DIRECTION('center_axis',(0.,0.,-1.));
#33381=DIRECTION('ref_axis',(0.707106781186548,0.707106781186547,0.));
#33382=DIRECTION('',(0.,-0.382683432365139,0.923879532511267));
#33383=DIRECTION('center_axis',(0.,0.,-1.));
#33384=DIRECTION('ref_axis',(0.707106781186548,0.707106781186547,0.));
#33385=DIRECTION('center_axis',(0.,0.,1.));
#33386=DIRECTION('ref_axis',(0.707106781186548,0.707106781186548,0.));
#33387=DIRECTION('center_axis',(0.,0.923879532511284,0.382683432365098));
#33388=DIRECTION('ref_axis',(0.,-0.382683432365098,0.923879532511284));
#33389=DIRECTION('',(0.,-0.382683432365073,0.923879532511294));
#33390=DIRECTION('',(1.,0.,0.));
#33391=DIRECTION('',(-1.,0.,0.));
#33392=DIRECTION('center_axis',(0.,0.,-1.));
#33393=DIRECTION('ref_axis',(-0.707106781186548,0.707106781186547,0.));
#33394=DIRECTION('',(0.382683432365135,0.,0.923879532511268));
#33395=DIRECTION('center_axis',(0.,0.,-1.));
#33396=DIRECTION('ref_axis',(-0.707106781186548,0.707106781186547,0.));
#33397=DIRECTION('center_axis',(0.,0.,1.));
#33398=DIRECTION('ref_axis',(-0.707106781186548,0.707106781186548,0.));
#33399=DIRECTION('center_axis',(-0.923879532511285,0.,0.382683432365094));
#33400=DIRECTION('ref_axis',(0.382683432365094,0.,0.923879532511285));
#33401=DIRECTION('',(0.382683432365069,0.,0.923879532511296));
#33402=DIRECTION('',(0.,1.,0.));
#33403=DIRECTION('',(0.,-1.,0.));
#33404=DIRECTION('center_axis',(0.,0.,-1.));
#33405=DIRECTION('ref_axis',(-0.707106781186548,-0.707106781186548,0.));
#33406=DIRECTION('center_axis',(0.,0.,1.));
#33407=DIRECTION('ref_axis',(-0.707106781186548,-0.707106781186548,0.));
#33408=DIRECTION('center_axis',(0.,0.,1.));
#33409=DIRECTION('ref_axis',(0.707106781186548,0.707106781186548,0.));
#33410=DIRECTION('',(0.,0.,-1.));
#33411=DIRECTION('center_axis',(0.,0.,-1.));
#33412=DIRECTION('ref_axis',(0.707106781186548,0.707106781186548,0.));
#33413=DIRECTION('',(0.,0.,1.));
#33414=DIRECTION('center_axis',(1.,0.,0.));
#33415=DIRECTION('ref_axis',(0.,1.,0.));
#33416=DIRECTION('',(0.,0.,1.));
#33417=DIRECTION('',(0.,-1.,0.));
#33418=DIRECTION('center_axis',(0.,0.,1.));
#33419=DIRECTION('ref_axis',(0.707106781186548,-0.707106781186548,0.));
#33420=DIRECTION('',(0.,0.,-1.));
#33421=DIRECTION('center_axis',(0.,0.,-1.));
#33422=DIRECTION('ref_axis',(0.707106781186548,-0.707106781186548,0.));
#33423=DIRECTION('center_axis',(0.,-1.,0.));
#33424=DIRECTION('ref_axis',(1.,0.,0.));
#33425=DIRECTION('',(0.,0.,1.));
#33426=DIRECTION('',(-1.,0.,0.));
#33427=DIRECTION('center_axis',(0.,-1.,0.));
#33428=DIRECTION('ref_axis',(0.,0.,1.));
#33429=DIRECTION('center_axis',(0.,0.,-1.));
#33430=DIRECTION('ref_axis',(-0.707106781186548,0.707106781186548,0.));
#33431=DIRECTION('',(0.,0.70710678118655,-0.707106781186545));
#33432=DIRECTION('',(-0.707106781186535,0.,-0.70710678118656));
#33433=DIRECTION('center_axis',(-0.70710678118656,0.,0.707106781186535));
#33434=DIRECTION('ref_axis',(0.707106781186535,0.,0.70710678118656));
#33435=DIRECTION('center_axis',(0.707106781186541,0.707106781186554,0.));
#33436=DIRECTION('ref_axis',(0.,0.,-1.));
#33437=DIRECTION('',(-0.707106781186554,0.707106781186541,0.));
#33438=DIRECTION('',(0.,0.,1.));
#33439=DIRECTION('',(0.707106781186554,-0.707106781186541,0.));
#33440=DIRECTION('',(0.,0.,-1.));
#33441=DIRECTION('center_axis',(0.,-1.,0.));
#33442=DIRECTION('ref_axis',(0.707106781186547,0.,0.707106781186547));
#33443=DIRECTION('',(0.,-0.707106781186667,0.707106781186428));
#33444=DIRECTION('center_axis',(0.,1.,0.));
#33445=DIRECTION('ref_axis',(0.707106781186548,0.,0.707106781186548));
#33446=DIRECTION('center_axis',(0.,-1.,0.));
#33447=DIRECTION('ref_axis',(0.707106781186548,0.,0.707106781186548));
#33448=DIRECTION('center_axis',(0.,0.707106781186529,0.707106781186566));
#33449=DIRECTION('ref_axis',(1.,0.,0.));
#33450=DIRECTION('',(0.,-0.707106781186566,0.707106781186529));
#33451=DIRECTION('',(1.,0.,0.));
#33452=DIRECTION('',(-1.,0.,0.));
#33453=DIRECTION('center_axis',(0.,-1.,0.));
#33454=DIRECTION('ref_axis',(-0.707106781186547,0.,0.707106781186547));
#33455=DIRECTION('',(-0.707106781186504,-0.707106781186592,0.));
#33456=DIRECTION('center_axis',(0.,1.,0.));
#33457=DIRECTION('ref_axis',(-0.707106781186548,0.,0.707106781186548));
#33458=DIRECTION('center_axis',(0.,-1.,0.));
#33459=DIRECTION('ref_axis',(-0.707106781186548,0.,0.707106781186548));
#33460=DIRECTION('center_axis',(-0.707106781186548,0.707106781186548,0.));
#33461=DIRECTION('ref_axis',(0.,0.,1.));
#33462=DIRECTION('',(-0.707106781186548,-0.707106781186548,0.));
#33463=DIRECTION('',(0.,0.,1.));
#33464=DIRECTION('',(0.,0.,-1.));
#33465=DIRECTION('center_axis',(0.,0.,1.));
#33466=DIRECTION('ref_axis',(1.,0.,0.));
#33467=DIRECTION('',(-1.,0.,0.));
#33468=DIRECTION('center_axis',(0.,0.,-1.));
#33469=DIRECTION('ref_axis',(1.,0.,0.));
#33470=DIRECTION('',(0.,-1.,0.));
#33471=DIRECTION('center_axis',(0.,1.,0.));
#33472=DIRECTION('ref_axis',(-1.,0.,0.));
#33473=DIRECTION('',(-1.,0.,0.));
#33474=DIRECTION('',(1.,0.,0.));
#33475=DIRECTION('center_axis',(-0.707106781186548,-0.707106781186548,0.));
#33476=DIRECTION('ref_axis',(0.,0.,1.));
#33477=DIRECTION('',(-0.707106781186548,0.707106781186548,0.));
#33478=DIRECTION('',(0.,0.,1.));
#33479=DIRECTION('',(-0.707106781186548,0.707106781186548,0.));
#33480=DIRECTION('',(0.,0.,-1.));
#33481=DIRECTION('center_axis',(0.,1.,0.));
#33482=DIRECTION('ref_axis',(-0.707106781186547,0.,0.707106781186547));
#33483=DIRECTION('',(0.,0.707106781186667,0.707106781186428));
#33484=DIRECTION('center_axis',(0.,-1.,0.));
#33485=DIRECTION('ref_axis',(-0.707106781186548,0.,0.707106781186548));
#33486=DIRECTION('center_axis',(0.,1.,0.));
#33487=DIRECTION('ref_axis',(-0.707106781186548,0.,0.707106781186548));
#33488=DIRECTION('center_axis',(0.,-0.707106781186529,0.707106781186566));
#33489=DIRECTION('ref_axis',(1.,0.,0.));
#33490=DIRECTION('',(0.,0.707106781186566,0.707106781186529));
#33491=DIRECTION('',(-1.,0.,0.));
#33492=DIRECTION('',(1.,0.,0.));
#33493=DIRECTION('center_axis',(0.,1.,0.));
#33494=DIRECTION('ref_axis',(0.707106781186547,0.,0.707106781186547));
#33495=DIRECTION('',(0.70710678118651,0.707106781186585,0.));
#33496=DIRECTION('center_axis',(0.,-1.,0.));
#33497=DIRECTION('ref_axis',(0.707106781186548,0.,0.707106781186548));
#33498=DIRECTION('center_axis',(0.,1.,0.));
#33499=DIRECTION('ref_axis',(0.707106781186548,0.,0.707106781186548));
#33500=DIRECTION('center_axis',(0.707106781186548,-0.707106781186548,0.));
#33501=DIRECTION('ref_axis',(0.,0.,-1.));
#33502=DIRECTION('',(-0.707106781186548,-0.707106781186548,0.));
#33503=DIRECTION('',(0.,0.,1.));
#33504=DIRECTION('',(0.,0.,-1.));
#33505=DIRECTION('center_axis',(0.,-1.,0.));
#33506=DIRECTION('ref_axis',(1.,0.,0.));
#33507=DIRECTION('',(-1.,0.,0.));
#33508=DIRECTION('center_axis',(0.,1.,0.));
#33509=DIRECTION('ref_axis',(1.,0.,0.));
#33510=DIRECTION('center_axis',(0.707106781186541,0.707106781186554,0.));
#33511=DIRECTION('ref_axis',(0.,0.,-1.));
#33512=DIRECTION('',(0.707106781186554,-0.707106781186541,0.));
#33513=DIRECTION('',(0.,0.,1.));
#33514=DIRECTION('',(0.707106781186554,-0.707106781186541,0.));
#33515=DIRECTION('',(0.,0.,-1.));
#33516=DIRECTION('center_axis',(0.,-1.,0.));
#33517=DIRECTION('ref_axis',(0.707106781186547,0.,0.707106781186547));
#33518=DIRECTION('',(0.,-0.707106781186667,0.707106781186428));
#33519=DIRECTION('center_axis',(0.,1.,0.));
#33520=DIRECTION('ref_axis',(0.707106781186548,0.,0.707106781186548));
#33521=DIRECTION('center_axis',(0.,-1.,0.));
#33522=DIRECTION('ref_axis',(0.707106781186548,0.,0.707106781186548));
#33523=DIRECTION('center_axis',(0.,0.707106781186529,0.707106781186566));
#33524=DIRECTION('ref_axis',(1.,0.,0.));
#33525=DIRECTION('',(0.,-0.707106781186566,0.707106781186529));
#33526=DIRECTION('',(1.,0.,0.));
#33527=DIRECTION('',(-1.,0.,0.));
#33528=DIRECTION('center_axis',(0.,-1.,0.));
#33529=DIRECTION('ref_axis',(-0.707106781186547,0.,0.707106781186547));
#33530=DIRECTION('',(-0.707106781186504,-0.707106781186592,0.));
#33531=DIRECTION('center_axis',(0.,1.,0.));
#33532=DIRECTION('ref_axis',(-0.707106781186548,0.,0.707106781186548));
#33533=DIRECTION('center_axis',(0.,-1.,0.));
#33534=DIRECTION('ref_axis',(-0.707106781186548,0.,0.707106781186548));
#33535=DIRECTION('center_axis',(-0.707106781186554,0.707106781186541,0.));
#33536=DIRECTION('ref_axis',(0.,0.,1.));
#33537=DIRECTION('',(0.707106781186541,0.707106781186554,0.));
#33538=DIRECTION('',(0.,0.,1.));
#33539=DIRECTION('',(0.,0.,-1.));
#33540=DIRECTION('center_axis',(0.,1.,0.));
#33541=DIRECTION('ref_axis',(-1.,0.,0.));
#33542=DIRECTION('',(1.,0.,0.));
#33543=DIRECTION('center_axis',(0.,-1.,0.));
#33544=DIRECTION('ref_axis',(1.,0.,0.));
#33545=DIRECTION('center_axis',(-0.707106781186548,-0.707106781186548,0.));
#33546=DIRECTION('ref_axis',(0.,0.,1.));
#33547=DIRECTION('',(0.707106781186548,-0.707106781186548,0.));
#33548=DIRECTION('',(0.,0.,1.));
#33549=DIRECTION('',(-0.707106781186548,0.707106781186548,0.));
#33550=DIRECTION('',(0.,0.,-1.));
#33551=DIRECTION('center_axis',(0.,1.,0.));
#33552=DIRECTION('ref_axis',(-0.707106781186547,0.,0.707106781186547));
#33553=DIRECTION('',(0.,0.707106781186667,0.707106781186428));
#33554=DIRECTION('center_axis',(0.,-1.,0.));
#33555=DIRECTION('ref_axis',(-0.707106781186548,0.,0.707106781186548));
#33556=DIRECTION('center_axis',(0.,1.,0.));
#33557=DIRECTION('ref_axis',(-0.707106781186548,0.,0.707106781186548));
#33558=DIRECTION('center_axis',(0.,-0.707106781186529,0.707106781186566));
#33559=DIRECTION('ref_axis',(1.,0.,0.));
#33560=DIRECTION('',(0.,0.707106781186566,0.707106781186529));
#33561=DIRECTION('',(-1.,0.,0.));
#33562=DIRECTION('',(1.,0.,0.));
#33563=DIRECTION('center_axis',(0.,1.,0.));
#33564=DIRECTION('ref_axis',(0.707106781186547,0.,0.707106781186547));
#33565=DIRECTION('',(0.70710678118651,0.707106781186585,0.));
#33566=DIRECTION('center_axis',(0.,-1.,0.));
#33567=DIRECTION('ref_axis',(0.707106781186548,0.,0.707106781186548));
#33568=DIRECTION('center_axis',(0.,1.,0.));
#33569=DIRECTION('ref_axis',(0.707106781186548,0.,0.707106781186548));
#33570=DIRECTION('center_axis',(0.707106781186548,-0.707106781186548,0.));
#33571=DIRECTION('ref_axis',(0.,0.,-1.));
#33572=DIRECTION('',(0.707106781186548,0.707106781186548,0.));
#33573=DIRECTION('',(0.,0.,1.));
#33574=DIRECTION('',(0.,0.,-1.));
#33575=DIRECTION('center_axis',(-1.,0.,0.));
#33576=DIRECTION('ref_axis',(0.,-1.,0.));
#33577=DIRECTION('',(0.,1.,0.));
#33578=DIRECTION('',(0.,-1.,0.));
#33579=DIRECTION('',(0.,-1.,0.));
#33580=DIRECTION('center_axis',(0.,-1.,0.));
#33581=DIRECTION('ref_axis',(-0.707106781186548,0.,0.707106781186548));
#33582=DIRECTION('',(0.,1.,0.));
#33583=DIRECTION('center_axis',(0.,0.,1.));
#33584=DIRECTION('ref_axis',(1.,0.,0.));
#33585=DIRECTION('',(0.,-1.,0.));
#33586=DIRECTION('center_axis',(0.,1.,0.));
#33587=DIRECTION('ref_axis',(0.707106781186548,0.,0.707106781186548));
#33588=DIRECTION('',(0.,1.,0.));
#33589=DIRECTION('center_axis',(1.,0.,0.));
#33590=DIRECTION('ref_axis',(0.,1.,0.));
#33591=DIRECTION('',(0.,1.,0.));
#33592=DIRECTION('',(0.,-1.,0.));
#33593=DIRECTION('center_axis',(0.,0.,1.));
#33594=DIRECTION('ref_axis',(1.,0.,0.));
#33595=DIRECTION('',(1.,0.,0.));
#33596=DIRECTION('center_axis',(0.,0.,-1.));
#33597=DIRECTION('ref_axis',(1.,0.,0.));
#33598=DIRECTION('center_axis',(0.,0.,-1.));
#33599=DIRECTION('ref_axis',(1.,0.,0.));
#33600=DIRECTION('center_axis',(0.,0.,-1.));
#33601=DIRECTION('ref_axis',(1.,0.,0.));
#33602=DIRECTION('',(-0.707106781186566,-8.65956056235516E-17,-0.707106781186529));
#33603=DIRECTION('center_axis',(0.,0.,1.));
#33604=DIRECTION('ref_axis',(1.,0.,0.));
#33605=DIRECTION('center_axis',(0.,0.,1.));
#33606=DIRECTION('ref_axis',(1.,0.,0.));
#33607=DIRECTION('center_axis',(0.,0.,1.));
#33608=DIRECTION('ref_axis',(1.,0.,0.));
#33609=DIRECTION('center_axis',(0.,0.,1.));
#33610=DIRECTION('ref_axis',(1.,0.,0.));
#33611=DIRECTION('',(0.,0.,-1.));
#33612=DIRECTION('center_axis',(0.,0.,1.));
#33613=DIRECTION('ref_axis',(1.,0.,0.));
#33614=DIRECTION('',(0.707106781186566,8.65956056235517E-17,-0.707106781186529));
#33615=DIRECTION('center_axis',(0.,0.,-1.));
#33616=DIRECTION('ref_axis',(1.,0.,0.));
#33617=DIRECTION('center_axis',(0.,0.,1.));
#33618=DIRECTION('ref_axis',(1.,0.,0.));
#33619=DIRECTION('center_axis',(0.,0.,1.));
#33620=DIRECTION('ref_axis',(1.,0.,0.));
#33621=DIRECTION('',(0.,0.,1.));
#33622=DIRECTION('center_axis',(0.,-1.,0.));
#33623=DIRECTION('ref_axis',(0.,0.,1.));
#33624=DIRECTION('',(-8.6595605623547E-17,0.707106781186566,0.707106781186529));
#33625=DIRECTION('center_axis',(0.,1.,0.));
#33626=DIRECTION('ref_axis',(0.,0.,1.));
#33627=DIRECTION('center_axis',(0.,1.,0.));
#33628=DIRECTION('ref_axis',(0.,0.,1.));
#33629=DIRECTION('',(0.,1.,0.));
#33630=DIRECTION('center_axis',(0.,1.,0.));
#33631=DIRECTION('ref_axis',(1.,0.,0.));
#33632=DIRECTION('center_axis',(0.,-1.,0.));
#33633=DIRECTION('ref_axis',(0.,0.,1.));
#33634=DIRECTION('',(1.04972719113862E-16,0.515038074910053,0.857167300702113));
#33635=DIRECTION('center_axis',(0.,0.,1.));
#33636=DIRECTION('ref_axis',(1.,0.,0.));
#33637=DIRECTION('',(-0.857167300702114,-1.04972719113862E-16,0.515038074910051));
#33638=DIRECTION('center_axis',(0.,1.,0.));
#33639=DIRECTION('ref_axis',(1.,0.,0.));
#33640=DIRECTION('',(0.,-1.,0.));
#33641=DIRECTION('center_axis',(0.,-1.,0.));
#33642=DIRECTION('ref_axis',(-0.707106781186548,0.,0.707106781186548));
#33643=DIRECTION('',(0.,-1.,0.));
#33644=DIRECTION('',(0.,1.,0.));
#33645=DIRECTION('center_axis',(0.,0.,1.));
#33646=DIRECTION('ref_axis',(1.,0.,0.));
#33647=DIRECTION('',(0.,-1.,0.));
#33648=DIRECTION('center_axis',(0.,1.,0.));
#33649=DIRECTION('ref_axis',(0.707106781186548,0.,0.707106781186548));
#33650=DIRECTION('',(0.,1.,0.));
#33651=DIRECTION('center_axis',(0.,0.,1.));
#33652=DIRECTION('ref_axis',(1.,0.,0.));
#33653=DIRECTION('',(0.,1.,0.));
#33654=DIRECTION('center_axis',(0.,0.,-1.));
#33655=DIRECTION('ref_axis',(1.,0.,0.));
#33656=DIRECTION('center_axis',(1.,0.,0.));
#33657=DIRECTION('ref_axis',(0.,1.,0.));
#33658=DIRECTION('',(0.,-1.,0.));
#33659=DIRECTION('center_axis',(-1.,0.,0.));
#33660=DIRECTION('ref_axis',(0.,-1.,0.));
#33661=DIRECTION('',(0.,1.,0.));
#33662=DIRECTION('center_axis',(0.,0.,1.));
#33663=DIRECTION('ref_axis',(1.,0.,0.));
#33664=DIRECTION('center_axis',(0.,0.,-1.));
#33665=DIRECTION('ref_axis',(1.,0.,0.));
#33666=DIRECTION('center_axis',(0.,0.,1.));
#33667=DIRECTION('ref_axis',(1.,0.,0.));
#33668=DIRECTION('center_axis',(0.,0.,-1.));
#33669=DIRECTION('ref_axis',(1.,0.,0.));
#33670=DIRECTION('',(1.,0.,0.));
#33671=DIRECTION('center_axis',(0.,-1.,0.));
#33672=DIRECTION('ref_axis',(1.,0.,0.));
#33673=DIRECTION('',(-1.,0.,0.));
#33674=DIRECTION('center_axis',(0.,0.,1.));
#33675=DIRECTION('ref_axis',(1.,0.,0.));
#33676=DIRECTION('center_axis',(0.,0.,-1.));
#33677=DIRECTION('ref_axis',(1.,0.,0.));
#33678=DIRECTION('center_axis',(0.,0.,1.));
#33679=DIRECTION('ref_axis',(1.,0.,0.));
#33680=DIRECTION('center_axis',(0.,0.,-1.));
#33681=DIRECTION('ref_axis',(1.,0.,0.));
#33682=DIRECTION('center_axis',(0.,0.,-1.));
#33683=DIRECTION('ref_axis',(1.,0.,0.));
#33684=DIRECTION('center_axis',(0.,0.,-1.));
#33685=DIRECTION('ref_axis',(1.,0.,0.));
#33686=DIRECTION('center_axis',(0.,0.,-1.));
#33687=DIRECTION('ref_axis',(1.,0.,0.));
#33688=DIRECTION('',(-0.707106781186535,-8.65956056235478E-17,-0.70710678118656));
#33689=DIRECTION('center_axis',(0.,0.,1.));
#33690=DIRECTION('ref_axis',(1.,0.,0.));
#33691=DIRECTION('center_axis',(0.,0.,1.));
#33692=DIRECTION('ref_axis',(1.,0.,0.));
#33693=DIRECTION('',(0.,0.,-1.));
#33694=DIRECTION('center_axis',(0.,0.,1.));
#33695=DIRECTION('ref_axis',(1.,0.,0.));
#33696=DIRECTION('center_axis',(0.,0.,1.));
#33697=DIRECTION('ref_axis',(1.,0.,0.));
#33698=DIRECTION('',(0.707106781186568,8.65956056235518E-17,-0.707106781186527));
#33699=DIRECTION('center_axis',(0.,0.,-1.));
#33700=DIRECTION('ref_axis',(1.,0.,0.));
#33701=DIRECTION('center_axis',(0.,0.,1.));
#33702=DIRECTION('ref_axis',(1.,0.,0.));
#33703=DIRECTION('center_axis',(0.,0.,1.));
#33704=DIRECTION('ref_axis',(1.,0.,0.));
#33705=DIRECTION('',(0.,0.,1.));
#33706=DIRECTION('center_axis',(0.,0.,1.));
#33707=DIRECTION('ref_axis',(1.,0.,0.));
#33708=DIRECTION('center_axis',(0.,0.,1.));
#33709=DIRECTION('ref_axis',(1.,0.,0.));
#33710=DIRECTION('center_axis',(0.,0.,1.));
#33711=DIRECTION('ref_axis',(1.,0.,0.));
#33712=DIRECTION('center_axis',(0.,0.,1.));
#33713=DIRECTION('ref_axis',(1.,0.,0.));
#33714=DIRECTION('center_axis',(0.,0.,-1.));
#33715=DIRECTION('ref_axis',(-1.,0.,0.));
#33716=DIRECTION('center_axis',(0.,0.,-1.));
#33717=DIRECTION('ref_axis',(1.,0.,0.));
#33718=DIRECTION('center_axis',(0.,0.,-1.));
#33719=DIRECTION('ref_axis',(-1.,0.,0.));
#33720=DIRECTION('center_axis',(0.,0.,-1.));
#33721=DIRECTION('ref_axis',(-1.,0.,0.));
#33722=DIRECTION('center_axis',(0.,0.,-1.));
#33723=DIRECTION('ref_axis',(1.,0.,0.));
#33724=DIRECTION('center_axis',(-1.22464679914735E-16,-1.,0.));
#33725=DIRECTION('ref_axis',(1.,-1.22464679914735E-16,0.));
#33726=DIRECTION('center_axis',(0.,0.,-1.));
#33727=DIRECTION('ref_axis',(1.,0.,0.));
#33728=DIRECTION('center_axis',(0.,0.,1.));
#33729=DIRECTION('ref_axis',(1.,0.,0.));
#33730=DIRECTION('center_axis',(0.,0.,1.));
#33731=DIRECTION('ref_axis',(1.,0.,0.));
#33732=DIRECTION('',(0.,0.,-1.));
#33733=DIRECTION('center_axis',(0.,0.,-1.));
#33734=DIRECTION('ref_axis',(-1.,0.,0.));
#33735=DIRECTION('center_axis',(0.,0.,1.));
#33736=DIRECTION('ref_axis',(1.,0.,0.));
#33737=DIRECTION('center_axis',(0.,0.,1.));
#33738=DIRECTION('ref_axis',(1.,0.,0.));
#33739=DIRECTION('center_axis',(0.,0.,1.));
#33740=DIRECTION('ref_axis',(1.,0.,0.));
#33741=DIRECTION('',(0.70710678118657,8.6595605623552E-17,-0.707106781186525));
#33742=DIRECTION('center_axis',(0.,0.,1.));
#33743=DIRECTION('ref_axis',(1.,0.,0.));
#33744=DIRECTION('center_axis',(0.,0.,1.));
#33745=DIRECTION('ref_axis',(1.,0.,0.));
#33746=DIRECTION('',(0.,0.,-1.));
#33747=DIRECTION('center_axis',(0.,0.,-1.));
#33748=DIRECTION('ref_axis',(1.,0.,0.));
#33749=DIRECTION('',(-0.70710678118657,-8.6595605623552E-17,-0.707106781186525));
#33750=DIRECTION('center_axis',(0.707106781186529,0.,-0.707106781186566));
#33751=DIRECTION('ref_axis',(-0.707106781186566,0.,-0.707106781186529));
#33752=DIRECTION('',(0.707106781186566,0.,0.707106781186529));
#33753=DIRECTION('',(-0.707106781186566,0.,-0.707106781186529));
#33754=DIRECTION('',(0.,1.,0.));
#33755=DIRECTION('center_axis',(0.,0.,1.));
#33756=DIRECTION('ref_axis',(0.707106781186547,0.707106781186547,0.));
#33757=DIRECTION('',(0.,0.707106781186566,0.707106781186529));
#33758=DIRECTION('center_axis',(0.,0.,1.));
#33759=DIRECTION('ref_axis',(0.707106781186548,0.707106781186548,0.));
#33760=DIRECTION('center_axis',(0.,0.707106781186529,-0.707106781186566));
#33761=DIRECTION('ref_axis',(-1.,0.,0.));
#33762=DIRECTION('',(0.,0.707106781186566,0.707106781186529));
#33763=DIRECTION('',(1.,0.,0.));
#33764=DIRECTION('',(-1.,0.,0.));
#33765=DIRECTION('center_axis',(0.,0.,1.));
#33766=DIRECTION('ref_axis',(-0.707106781186547,0.707106781186547,0.));
#33767=DIRECTION('',(-0.707106781186573,0.,0.707106781186522));
#33768=DIRECTION('center_axis',(0.,0.,-1.));
#33769=DIRECTION('ref_axis',(-0.707106781186548,0.707106781186548,0.));
#33770=DIRECTION('center_axis',(0.,0.,1.));
#33771=DIRECTION('ref_axis',(-0.707106781186548,0.707106781186548,0.));
#33772=DIRECTION('center_axis',(-0.707106781186529,0.,-0.707106781186566));
#33773=DIRECTION('ref_axis',(-0.707106781186566,0.,0.707106781186529));
#33774=DIRECTION('',(-0.707106781186566,0.,0.707106781186529));
#33775=DIRECTION('',(0.,1.,0.));
#33776=DIRECTION('',(0.,-1.,0.));
#33777=DIRECTION('center_axis',(0.,0.,1.));
#33778=DIRECTION('ref_axis',(-0.707106781186547,-0.707106781186547,0.));
#33779=DIRECTION('',(0.,-0.707106781186573,0.707106781186522));
#33780=DIRECTION('center_axis',(0.,0.,-1.));
#33781=DIRECTION('ref_axis',(-0.707106781186548,-0.707106781186548,0.));
#33782=DIRECTION('center_axis',(0.,0.,1.));
#33783=DIRECTION('ref_axis',(-0.707106781186548,-0.707106781186548,0.));
#33784=DIRECTION('center_axis',(0.,-0.707106781186529,-0.707106781186566));
#33785=DIRECTION('ref_axis',(-1.,0.,0.));
#33786=DIRECTION('',(0.,-0.707106781186566,0.707106781186529));
#33787=DIRECTION('',(1.,0.,0.));
#33788=DIRECTION('center_axis',(0.,0.,1.));
#33789=DIRECTION('ref_axis',(0.707106781186547,-0.707106781186547,0.));
#33790=DIRECTION('center_axis',(0.,0.,1.));
#33791=DIRECTION('ref_axis',(0.707106781186548,-0.707106781186548,0.));
#33792=DIRECTION('center_axis',(0.,0.,1.));
#33793=DIRECTION('ref_axis',(-0.707106781186548,-0.707106781186548,0.));
#33794=DIRECTION('',(0.,0.,-1.));
#33795=DIRECTION('center_axis',(0.,0.,1.));
#33796=DIRECTION('ref_axis',(1.,0.,0.));
#33797=DIRECTION('center_axis',(0.,0.707106781186561,0.707106781186534));
#33798=DIRECTION('ref_axis',(1.,0.,0.));
#33799=DIRECTION('',(0.,0.707106781186534,-0.707106781186561));
#33800=DIRECTION('center_axis',(0.,0.,-1.));
#33801=DIRECTION('ref_axis',(0.707106781186548,0.707106781186548,0.));
#33802=DIRECTION('center_axis',(-1.,0.,0.));
#33803=DIRECTION('ref_axis',(0.,-1.,0.));
#33804=DIRECTION('',(0.,0.,1.));
#33805=DIRECTION('center_axis',(0.,0.,1.));
#33806=DIRECTION('ref_axis',(-0.707106781186548,0.707106781186548,0.));
#33807=DIRECTION('',(0.,0.,-1.));
#33808=DIRECTION('center_axis',(0.,1.,0.));
#33809=DIRECTION('ref_axis',(-1.,0.,0.));
#43529=CARTESIAN_POINT('',(0.,0.,0.));
#43530=CARTESIAN_POINT('Origin',(-9.5,-8.5,109.464644660941));
#43531=CARTESIAN_POINT('',(-10.1,-8.5,109.5));
#43532=CARTESIAN_POINT('',(-10.2707106781187,-8.5,109.429289321881));
#43533=CARTESIAN_POINT('',(-10.1,-8.5,109.5));
#43534=CARTESIAN_POINT('',(-9.5,-9.27071067811865,109.429289321881));
#43535=CARTESIAN_POINT('Origin',(-9.5,-8.5,109.429289321881));
#43536=CARTESIAN_POINT('',(-9.5,-9.1,109.5));
#43537=CARTESIAN_POINT('',(-9.5,-9.27071067811865,109.429289321881));
#43538=CARTESIAN_POINT('Origin',(-9.5,-8.5,109.5));
#43539=CARTESIAN_POINT('Origin',(-10.1853553390593,0.8125,109.464644660941));
#43540=CARTESIAN_POINT('',(-10.1,6.,109.5));
#43541=CARTESIAN_POINT('',(-10.2707106781187,6.,109.429289321881));
#43542=CARTESIAN_POINT('',(-10.1,6.,109.5));
#43543=CARTESIAN_POINT('',(-10.2707106781187,0.8125,109.429289321881));
#43544=CARTESIAN_POINT('',(-10.1,0.8125,109.5));
#43545=CARTESIAN_POINT('Origin',(-9.5,6.,109.464644660941));
#43546=CARTESIAN_POINT('',(-9.5,6.6,109.5));
#43547=CARTESIAN_POINT('',(-9.5,6.77071067811865,109.429289321881));
#43548=CARTESIAN_POINT('',(-9.5,6.6,109.5));
#43549=CARTESIAN_POINT('Origin',(-9.5,6.,109.429289321881));
#43550=CARTESIAN_POINT('Origin',(-9.5,6.,109.5));
#43551=CARTESIAN_POINT('Origin',(2.625,6.68535533905934,109.464644660941));
#43552=CARTESIAN_POINT('',(9.5,6.60000000000001,109.5));
#43553=CARTESIAN_POINT('',(9.5,6.77071067811867,109.429289321881));
#43554=CARTESIAN_POINT('',(9.5,6.60000000000001,109.5));
#43555=CARTESIAN_POINT('',(2.625,6.77071067811866,109.429289321881));
#43556=CARTESIAN_POINT('',(2.625,6.60000000000001,109.5));
#43557=CARTESIAN_POINT('Origin',(9.5,6.,109.464644660941));
#43558=CARTESIAN_POINT('',(10.1,6.,109.5));
#43559=CARTESIAN_POINT('',(10.2707106781187,6.,109.429289321881));
#43560=CARTESIAN_POINT('',(10.1,6.,109.5));
#43561=CARTESIAN_POINT('Origin',(9.5,6.,109.429289321881));
#43562=CARTESIAN_POINT('Origin',(9.5,6.,109.5));
#43563=CARTESIAN_POINT('Origin',(10.1853553390593,-3.3125,109.464644660941));
#43564=CARTESIAN_POINT('',(10.1,-8.5,109.5));
#43565=CARTESIAN_POINT('',(10.2707106781187,-8.5,109.429289321881));
#43566=CARTESIAN_POINT('',(10.1,-8.5,109.5));
#43567=CARTESIAN_POINT('',(10.2707106781187,-3.3125,109.429289321881));
#43568=CARTESIAN_POINT('',(10.1,-3.3125,109.5));
#43569=CARTESIAN_POINT('Origin',(9.5,-8.5,109.464644660941));
#43570=CARTESIAN_POINT('',(9.5,-9.1,109.5));
#43571=CARTESIAN_POINT('',(9.5,-9.27071067811865,109.429289321881));
#43572=CARTESIAN_POINT('',(9.5,-9.1,109.5));
#43573=CARTESIAN_POINT('Origin',(9.5,-8.5,109.429289321881));
#43574=CARTESIAN_POINT('Origin',(9.5,-8.5,109.5));
#43575=CARTESIAN_POINT('Origin',(-2.625,-9.18535533905934,109.464644660941));
#43576=CARTESIAN_POINT('',(-2.625,-9.27071067811866,109.429289321881));
#43577=CARTESIAN_POINT('',(-2.625,-9.10000000000001,109.5));
#43578=CARTESIAN_POINT('Origin',(10.35,-5.375,109.35));
#43579=CARTESIAN_POINT('',(10.4292893218813,-8.5,109.270710678119));
#43580=CARTESIAN_POINT('',(10.2,-8.5,109.5));
#43581=CARTESIAN_POINT('',(10.4292893218814,6.,109.270710678119));
#43582=CARTESIAN_POINT('',(10.4292893218813,-7.4375,109.270710678119));
#43583=CARTESIAN_POINT('',(10.2,6.,109.5));
#43584=CARTESIAN_POINT('Origin',(9.5,-8.5,109.35));
#43585=CARTESIAN_POINT('',(9.5,-9.42928932188135,109.270710678119));
#43586=CARTESIAN_POINT('',(9.5,-9.2,109.5));
#43587=CARTESIAN_POINT('Origin',(9.5,-8.5,109.270710678119));
#43588=CARTESIAN_POINT('Origin',(-5.25,-9.35,109.35));
#43589=CARTESIAN_POINT('',(-9.5,-9.42928932188135,109.270710678119));
#43590=CARTESIAN_POINT('',(-9.5,-9.5,109.2));
#43591=CARTESIAN_POINT('',(-7.875,-9.42928932188135,109.270710678119));
#43592=CARTESIAN_POINT('Origin',(-9.5,-8.5,109.35));
#43593=CARTESIAN_POINT('',(-10.4292893218814,-8.5,109.270710678119));
#43594=CARTESIAN_POINT('',(-10.2,-8.5,109.5));
#43595=CARTESIAN_POINT('Origin',(-9.5,-8.5,109.270710678119));
#43596=CARTESIAN_POINT('Origin',(0.,-1.25,109.5));
#43597=CARTESIAN_POINT('',(5.4,-6.61309271539571E-16,109.5));
#43598=CARTESIAN_POINT('Origin',(0.,0.,109.5));
#43599=CARTESIAN_POINT('',(5.2,-7.2,109.5));
#43600=CARTESIAN_POINT('Origin',(7.,-7.2,109.5));
#43601=CARTESIAN_POINT('',(-9.5,1.22464679914735E-16,109.5));
#43602=CARTESIAN_POINT('Origin',(-8.5,0.,109.5));
#43603=CARTESIAN_POINT('Origin',(4.9545806272857,0.211749997425753,118.45));
#43604=CARTESIAN_POINT('',(4.99451026031136,0.23423761364175,124.9));
#43605=CARTESIAN_POINT('',(4.91465099426005,0.189262381209757,124.9));
#43606=CARTESIAN_POINT('',(4.869612960617,0.163897810114468,124.9));
#43607=CARTESIAN_POINT('',(4.91465099426005,0.189262381209757,124.5));
#43608=CARTESIAN_POINT('',(4.91465099426005,0.189262381209757,118.45));
#43609=CARTESIAN_POINT('',(4.99451026031136,0.23423761364175,124.5));
#43610=CARTESIAN_POINT('',(4.94553313233032,0.206654618909699,124.5));
#43611=CARTESIAN_POINT('',(4.99451026031136,0.23423761364175,118.45));
#43612=CARTESIAN_POINT('Origin',(4.85,0.,124.7));
#43613=CARTESIAN_POINT('',(4.91465099426005,-0.189262381209757,124.9));
#43614=CARTESIAN_POINT('Origin',(4.85,0.,124.9));
#43615=CARTESIAN_POINT('',(4.91465099426005,-0.189262381209757,124.5));
#43616=CARTESIAN_POINT('',(4.91465099426005,-0.189262381209757,118.45));
#43617=CARTESIAN_POINT('Origin',(4.85,0.,124.5));
#43618=CARTESIAN_POINT('Origin',(4.9545806272857,-0.211749997425753,118.45));
#43619=CARTESIAN_POINT('',(4.99451026031136,-0.23423761364175,124.5));
#43620=CARTESIAN_POINT('',(4.94553313233032,-0.206654618909699,124.5));
#43621=CARTESIAN_POINT('',(4.99451026031136,-0.23423761364175,124.9));
#43622=CARTESIAN_POINT('',(4.869612960617,-0.163897810114468,124.9));
#43623=CARTESIAN_POINT('',(4.99451026031136,-0.23423761364175,118.45));
#43624=CARTESIAN_POINT('Origin',(-7.875,-9.46464466094067,109.185355339059));
#43625=CARTESIAN_POINT('',(9.5,-9.5,109.1));
#43626=CARTESIAN_POINT('',(9.5,-9.5,109.1));
#43627=CARTESIAN_POINT('',(-9.5,-9.5,109.1));
#43628=CARTESIAN_POINT('',(-9.5,-9.42928932188135,109.270710678119));
#43629=CARTESIAN_POINT('',(-7.875,-9.5,109.1));
#43630=CARTESIAN_POINT('Origin',(9.5,-8.5,109.185355339059));
#43631=CARTESIAN_POINT('',(10.5,-8.5,109.1));
#43632=CARTESIAN_POINT('',(10.5,-8.5,109.1));
#43633=CARTESIAN_POINT('Origin',(9.5,-8.5,109.1));
#43634=CARTESIAN_POINT('Origin',(10.4646446609407,-7.4375,109.185355339059));
#43635=CARTESIAN_POINT('',(10.5,6.,109.1));
#43636=CARTESIAN_POINT('',(10.5,6.,109.1));
#43637=CARTESIAN_POINT('',(10.5,-7.4375,109.1));
#43638=CARTESIAN_POINT('Origin',(9.5,6.,109.185355339059));
#43639=CARTESIAN_POINT('',(9.5,7.,109.1));
#43640=CARTESIAN_POINT('',(9.5,6.92928932188134,109.270710678119));
#43641=CARTESIAN_POINT('',(9.5,7.,109.1));
#43642=CARTESIAN_POINT('Origin',(9.5,6.,109.270710678119));
#43643=CARTESIAN_POINT('Origin',(9.5,6.,109.1));
#43644=CARTESIAN_POINT('Origin',(7.875,6.96464466094067,109.185355339059));
#43645=CARTESIAN_POINT('',(-9.5,7.,109.1));
#43646=CARTESIAN_POINT('',(-9.5,6.92928932188135,109.270710678119));
#43647=CARTESIAN_POINT('',(-9.5,7.,109.1));
#43648=CARTESIAN_POINT('',(7.875,6.92928932188134,109.270710678119));
#43649=CARTESIAN_POINT('',(7.875,7.,109.1));
#43650=CARTESIAN_POINT('Origin',(-9.5,6.,109.185355339059));
#43651=CARTESIAN_POINT('',(-10.5,6.,109.1));
#43652=CARTESIAN_POINT('',(-10.4292893218813,6.,109.270710678119));
#43653=CARTESIAN_POINT('',(-10.5,6.,109.1));
#43654=CARTESIAN_POINT('Origin',(-9.5,6.,109.270710678119));
#43655=CARTESIAN_POINT('Origin',(-9.5,6.,109.1));
#43656=CARTESIAN_POINT('Origin',(-10.4646446609407,4.9375,109.185355339059));
#43657=CARTESIAN_POINT('',(-10.5,-8.5,109.1));
#43658=CARTESIAN_POINT('',(-10.5,-8.5,109.1));
#43659=CARTESIAN_POINT('',(-10.4292893218813,4.9375,109.270710678119));
#43660=CARTESIAN_POINT('',(-10.5,4.9375,109.1));
#43661=CARTESIAN_POINT('Origin',(-9.5,-8.5,109.185355339059));
#43662=CARTESIAN_POINT('Origin',(-9.5,-8.5,109.1));
#43663=CARTESIAN_POINT('Origin',(9.5,6.,107.));
#43664=CARTESIAN_POINT('',(10.5,6.,107.1));
#43665=CARTESIAN_POINT('',(10.5,6.,107.));
#43666=CARTESIAN_POINT('',(9.5,7.,107.1));
#43667=CARTESIAN_POINT('Origin',(9.5,6.,107.1));
#43668=CARTESIAN_POINT('',(9.5,7.,107.));
#43669=CARTESIAN_POINT('Origin',(10.5,-9.5,107.));
#43670=CARTESIAN_POINT('',(10.5,-8.5,107.1));
#43671=CARTESIAN_POINT('',(10.5,-8.5,107.));
#43672=CARTESIAN_POINT('',(10.5,-5.375,107.1));
#43673=CARTESIAN_POINT('Origin',(9.5,-8.5,107.));
#43674=CARTESIAN_POINT('',(9.5,-9.5,107.1));
#43675=CARTESIAN_POINT('',(9.5,-9.5,107.));
#43676=CARTESIAN_POINT('Origin',(9.5,-8.5,107.1));
#43677=CARTESIAN_POINT('Origin',(-10.5,-9.5,107.));
#43678=CARTESIAN_POINT('',(-9.5,-9.5,107.1));
#43679=CARTESIAN_POINT('',(-9.5,-9.5,107.));
#43680=CARTESIAN_POINT('',(-5.25,-9.5,107.1));
#43681=CARTESIAN_POINT('',(3.,-9.5,107.745));
#43682=CARTESIAN_POINT('Origin',(3.,-9.5,108.25));
#43683=CARTESIAN_POINT('Origin',(-9.5,6.,109.35));
#43684=CARTESIAN_POINT('',(-9.5,6.7,109.5));
#43685=CARTESIAN_POINT('',(-10.2,6.,109.5));
#43686=CARTESIAN_POINT('Origin',(-10.35,2.875,109.35));
#43687=CARTESIAN_POINT('Origin',(8.15,-5.8,123.5));
#43688=CARTESIAN_POINT('',(8.2,-5.85,123.5));
#43689=CARTESIAN_POINT('',(8.1,-5.75,123.5));
#43690=CARTESIAN_POINT('',(7.92499999999999,-5.575,123.5));
#43691=CARTESIAN_POINT('',(8.1,-5.75,128.));
#43692=CARTESIAN_POINT('',(8.1,-5.75,123.5));
#43693=CARTESIAN_POINT('',(8.2,-5.85,128.));
#43694=CARTESIAN_POINT('',(8.1,-5.75,128.));
#43695=CARTESIAN_POINT('',(8.2,-5.85,123.5));
#43696=CARTESIAN_POINT('Origin',(7.7,-5.8,128.));
#43697=CARTESIAN_POINT('',(7.7,-5.75,128.4));
#43698=CARTESIAN_POINT('',(7.7,-5.85,128.5));
#43699=CARTESIAN_POINT('',(7.7,-5.75,128.4));
#43700=CARTESIAN_POINT('Origin',(7.7,-5.85,128.));
#43701=CARTESIAN_POINT('Origin',(7.7,-5.75,128.));
#43702=CARTESIAN_POINT('Origin',(7.6,-5.8,128.45));
#43703=CARTESIAN_POINT('',(6.3,-5.75,128.4));
#43704=CARTESIAN_POINT('',(6.3,-5.85,128.5));
#43705=CARTESIAN_POINT('',(6.3,-5.75,128.4));
#43706=CARTESIAN_POINT('',(7.6,-5.85,128.5));
#43707=CARTESIAN_POINT('',(7.6,-5.75,128.4));
#43708=CARTESIAN_POINT('Origin',(6.3,-5.8,128.));
#43709=CARTESIAN_POINT('',(5.89999999999999,-5.75,128.));
#43710=CARTESIAN_POINT('',(5.8,-5.85,128.));
#43711=CARTESIAN_POINT('',(5.89999999999999,-5.75,128.));
#43712=CARTESIAN_POINT('Origin',(6.3,-5.85,128.));
#43713=CARTESIAN_POINT('Origin',(6.3,-5.75,128.));
#43714=CARTESIAN_POINT('Origin',(5.85,-5.8,123.5));
#43715=CARTESIAN_POINT('',(5.9,-5.75,123.5));
#43716=CARTESIAN_POINT('',(5.8,-5.85,123.5));
#43717=CARTESIAN_POINT('',(6.075,-5.575,123.5));
#43718=CARTESIAN_POINT('',(5.8,-5.85,123.5));
#43719=CARTESIAN_POINT('',(5.9,-5.75,123.5));
#43720=CARTESIAN_POINT('Origin',(7.,-6.05,123.5));
#43721=CARTESIAN_POINT('',(6.21259921259882,-5.75,123.5));
#43722=CARTESIAN_POINT('',(8.2,-5.75,123.5));
#43723=CARTESIAN_POINT('',(5.8,-6.06752483470939,123.5));
#43724=CARTESIAN_POINT('Origin',(7.,-7.2,123.5));
#43725=CARTESIAN_POINT('',(5.8,-5.75,123.5));
#43726=CARTESIAN_POINT('Origin',(8.2,-5.75,123.5));
#43727=CARTESIAN_POINT('',(7.78740078740118,-5.75,123.5));
#43728=CARTESIAN_POINT('',(8.2,-5.75,123.5));
#43729=CARTESIAN_POINT('',(7.6,-5.75,123.5));
#43730=CARTESIAN_POINT('Origin',(5.85,-6.3,123.5));
#43731=CARTESIAN_POINT('',(5.8,-6.25,123.5));
#43732=CARTESIAN_POINT('',(5.9,-6.35,123.5));
#43733=CARTESIAN_POINT('',(6.3625,-6.8125,123.5));
#43734=CARTESIAN_POINT('',(5.9,-6.35,128.));
#43735=CARTESIAN_POINT('',(5.9,-6.35,123.5));
#43736=CARTESIAN_POINT('',(5.8,-6.25,128.));
#43737=CARTESIAN_POINT('',(5.9,-6.35,128.));
#43738=CARTESIAN_POINT('',(5.8,-6.25,123.5));
#43739=CARTESIAN_POINT('Origin',(6.3,-6.3,128.));
#43740=CARTESIAN_POINT('',(6.3,-6.35,128.4));
#43741=CARTESIAN_POINT('',(6.3,-6.25,128.5));
#43742=CARTESIAN_POINT('',(6.3,-6.35,128.4));
#43743=CARTESIAN_POINT('Origin',(6.3,-6.25,128.));
#43744=CARTESIAN_POINT('Origin',(6.3,-6.35,128.));
#43745=CARTESIAN_POINT('Origin',(6.4,-6.3,128.45));
#43746=CARTESIAN_POINT('',(7.7,-6.35,128.4));
#43747=CARTESIAN_POINT('',(7.7,-6.25,128.5));
#43748=CARTESIAN_POINT('',(7.7,-6.35,128.4));
#43749=CARTESIAN_POINT('',(6.4,-6.25,128.5));
#43750=CARTESIAN_POINT('',(6.4,-6.35,128.4));
#43751=CARTESIAN_POINT('Origin',(7.7,-6.3,128.));
#43752=CARTESIAN_POINT('',(8.10000000000001,-6.35,128.));
#43753=CARTESIAN_POINT('',(8.2,-6.25,128.));
#43754=CARTESIAN_POINT('',(8.10000000000001,-6.35,128.));
#43755=CARTESIAN_POINT('Origin',(7.7,-6.25,128.));
#43756=CARTESIAN_POINT('Origin',(7.7,-6.35,128.));
#43757=CARTESIAN_POINT('Origin',(8.15,-6.3,123.5));
#43758=CARTESIAN_POINT('',(8.1,-6.35,123.5));
#43759=CARTESIAN_POINT('',(8.2,-6.25,123.5));
#43760=CARTESIAN_POINT('',(7.6375,-6.8125,123.5));
#43761=CARTESIAN_POINT('',(8.2,-6.25,123.5));
#43762=CARTESIAN_POINT('',(8.1,-6.35,123.5));
#43763=CARTESIAN_POINT('Origin',(5.8,-6.35,123.5));
#43764=CARTESIAN_POINT('',(6.4,-6.35,123.5));
#43765=CARTESIAN_POINT('',(6.5,-6.35,127.));
#43766=CARTESIAN_POINT('Origin',(7.,-6.35,127.));
#43767=CARTESIAN_POINT('Origin',(8.15,-8.1,123.5));
#43768=CARTESIAN_POINT('',(8.2,-8.15,123.5));
#43769=CARTESIAN_POINT('',(8.1,-8.05,123.5));
#43770=CARTESIAN_POINT('',(7.63749999999999,-7.58750000000001,123.5));
#43771=CARTESIAN_POINT('',(8.1,-8.05,128.));
#43772=CARTESIAN_POINT('',(8.1,-8.05,123.5));
#43773=CARTESIAN_POINT('',(8.2,-8.15,128.));
#43774=CARTESIAN_POINT('',(8.1,-8.05,128.));
#43775=CARTESIAN_POINT('',(8.2,-8.15,123.5));
#43776=CARTESIAN_POINT('Origin',(7.7,-8.1,128.));
#43777=CARTESIAN_POINT('',(7.7,-8.05,128.4));
#43778=CARTESIAN_POINT('',(7.7,-8.15,128.5));
#43779=CARTESIAN_POINT('',(7.7,-8.05,128.4));
#43780=CARTESIAN_POINT('Origin',(7.7,-8.15,128.));
#43781=CARTESIAN_POINT('Origin',(7.7,-8.05,128.));
#43782=CARTESIAN_POINT('Origin',(7.6,-8.1,128.45));
#43783=CARTESIAN_POINT('',(6.3,-8.05,128.4));
#43784=CARTESIAN_POINT('',(6.3,-8.15,128.5));
#43785=CARTESIAN_POINT('',(6.3,-8.05,128.4));
#43786=CARTESIAN_POINT('',(7.6,-8.15,128.5));
#43787=CARTESIAN_POINT('',(7.6,-8.05,128.4));
#43788=CARTESIAN_POINT('Origin',(6.3,-8.1,128.));
#43789=CARTESIAN_POINT('',(5.89999999999999,-8.05,128.));
#43790=CARTESIAN_POINT('',(5.8,-8.15,128.));
#43791=CARTESIAN_POINT('',(5.89999999999999,-8.05,128.));
#43792=CARTESIAN_POINT('Origin',(6.3,-8.15,128.));
#43793=CARTESIAN_POINT('Origin',(6.3,-8.05,128.));
#43794=CARTESIAN_POINT('Origin',(5.85,-8.1,123.5));
#43795=CARTESIAN_POINT('',(5.9,-8.05,123.5));
#43796=CARTESIAN_POINT('',(5.8,-8.15,123.5));
#43797=CARTESIAN_POINT('',(6.3625,-7.5875,123.5));
#43798=CARTESIAN_POINT('',(5.8,-8.15,123.5));
#43799=CARTESIAN_POINT('',(5.9,-8.05,123.5));
#43800=CARTESIAN_POINT('Origin',(8.2,-8.05,123.5));
#43801=CARTESIAN_POINT('',(7.6,-8.05,123.5));
#43802=CARTESIAN_POINT('',(6.5,-8.05,127.));
#43803=CARTESIAN_POINT('Origin',(7.,-8.05,127.));
#43804=CARTESIAN_POINT('Origin',(5.85,-8.6,123.5));
#43805=CARTESIAN_POINT('',(5.8,-8.55,123.5));
#43806=CARTESIAN_POINT('',(5.9,-8.65,123.5));
#43807=CARTESIAN_POINT('',(6.075,-8.825,123.5));
#43808=CARTESIAN_POINT('',(5.9,-8.65,128.));
#43809=CARTESIAN_POINT('',(5.9,-8.65,123.5));
#43810=CARTESIAN_POINT('',(5.8,-8.55,128.));
#43811=CARTESIAN_POINT('',(5.9,-8.65,128.));
#43812=CARTESIAN_POINT('',(5.8,-8.55,123.5));
#43813=CARTESIAN_POINT('Origin',(6.3,-8.6,128.));
#43814=CARTESIAN_POINT('',(6.3,-8.65,128.4));
#43815=CARTESIAN_POINT('',(6.3,-8.55,128.5));
#43816=CARTESIAN_POINT('',(6.3,-8.65,128.4));
#43817=CARTESIAN_POINT('Origin',(6.3,-8.55,128.));
#43818=CARTESIAN_POINT('Origin',(6.3,-8.65,128.));
#43819=CARTESIAN_POINT('Origin',(6.4,-8.6,128.45));
#43820=CARTESIAN_POINT('',(7.7,-8.65,128.4));
#43821=CARTESIAN_POINT('',(7.7,-8.55,128.5));
#43822=CARTESIAN_POINT('',(7.7,-8.65,128.4));
#43823=CARTESIAN_POINT('',(6.4,-8.55,128.5));
#43824=CARTESIAN_POINT('',(6.4,-8.65,128.4));
#43825=CARTESIAN_POINT('Origin',(7.7,-8.6,128.));
#43826=CARTESIAN_POINT('',(8.10000000000001,-8.65,128.));
#43827=CARTESIAN_POINT('',(8.2,-8.55,128.));
#43828=CARTESIAN_POINT('',(8.10000000000001,-8.65,128.));
#43829=CARTESIAN_POINT('Origin',(7.7,-8.55,128.));
#43830=CARTESIAN_POINT('Origin',(7.7,-8.65,128.));
#43831=CARTESIAN_POINT('Origin',(8.15,-8.6,123.5));
#43832=CARTESIAN_POINT('',(8.1,-8.65,123.5));
#43833=CARTESIAN_POINT('',(8.2,-8.55,123.5));
#43834=CARTESIAN_POINT('',(7.925,-8.825,123.5));
#43835=CARTESIAN_POINT('',(8.2,-8.55,123.5));
#43836=CARTESIAN_POINT('',(8.1,-8.65,123.5));
#43837=CARTESIAN_POINT('Origin',(5.8,-8.05,123.5));
#43838=CARTESIAN_POINT('',(5.8,-8.33247516529063,123.5));
#43839=CARTESIAN_POINT('',(5.8,-7.625,123.5));
#43840=CARTESIAN_POINT('',(5.8,-8.05,123.5));
#43841=CARTESIAN_POINT('',(5.8,-8.2,128.));
#43842=CARTESIAN_POINT('Origin',(6.3,-8.2,128.));
#43843=CARTESIAN_POINT('',(6.3,-8.2,128.5));
#43844=CARTESIAN_POINT('Origin',(7.,-8.35,128.5));
#43845=CARTESIAN_POINT('',(7.7,-8.5,128.5));
#43846=CARTESIAN_POINT('Origin',(7.7,-8.5,128.));
#43847=CARTESIAN_POINT('',(8.2,-8.5,128.));
#43848=CARTESIAN_POINT('Origin',(8.2,-8.65,123.5));
#43849=CARTESIAN_POINT('',(8.2,-8.33247516529064,123.5));
#43850=CARTESIAN_POINT('',(8.2,-8.65,123.5));
#43851=CARTESIAN_POINT('',(8.2,-7.925,123.5));
#43852=CARTESIAN_POINT('Origin',(7.,-8.35,123.5));
#43853=CARTESIAN_POINT('',(7.78740078740121,-8.65,123.5));
#43854=CARTESIAN_POINT('',(5.8,-8.65,123.5));
#43855=CARTESIAN_POINT('Origin',(7.,-7.2,123.5));
#43856=CARTESIAN_POINT('Origin',(-8.5,0.,110.45));
#43857=CARTESIAN_POINT('',(-9.4,1.10218211923262E-16,110.5));
#43858=CARTESIAN_POINT('Origin',(-8.5,0.,110.5));
#43859=CARTESIAN_POINT('',(-9.5,-1.22464679914735E-16,110.4));
#43860=CARTESIAN_POINT('',(-9.45,-1.16341445918999E-16,110.45));
#43861=CARTESIAN_POINT('Origin',(-8.5,0.,110.4));
#43862=CARTESIAN_POINT('Origin',(-8.5,0.,110.5));
#43863=CARTESIAN_POINT('',(-9.01,-6.2456986756515E-17,110.5));
#43864=CARTESIAN_POINT('Origin',(-8.5,0.,110.5));
#43865=CARTESIAN_POINT('Origin',(-8.5,0.,109.4));
#43866=CARTESIAN_POINT('',(-9.5,-1.22464679914735E-16,109.4));
#43867=CARTESIAN_POINT('Origin',(-8.5,0.,110.45));
#43868=CARTESIAN_POINT('',(-8.91,5.02105187650415E-17,110.4));
#43869=CARTESIAN_POINT('',(-8.96,-5.63337527607782E-17,110.45));
#43870=CARTESIAN_POINT('Origin',(-8.5,0.,110.4));
#43871=CARTESIAN_POINT('Origin',(-8.5,0.,110.115));
#43872=CARTESIAN_POINT('',(-8.91,-5.02105187650415E-17,109.7));
#43873=CARTESIAN_POINT('Origin',(-8.5,0.,109.7));
#43874=CARTESIAN_POINT('',(-8.91,-5.02105187650415E-17,110.115));
#43875=CARTESIAN_POINT('Origin',(3.,-9.45,108.25));
#43876=CARTESIAN_POINT('',(3.,-9.4,107.845));
#43877=CARTESIAN_POINT('',(3.,-9.45,107.795));
#43878=CARTESIAN_POINT('Origin',(3.,-9.4,108.25));
#43879=CARTESIAN_POINT('Origin',(3.,-8.515,108.25));
#43880=CARTESIAN_POINT('',(3.,-7.5,107.845));
#43881=CARTESIAN_POINT('',(3.,-8.515,107.845));
#43882=CARTESIAN_POINT('Origin',(3.,-7.5,108.25));
#43883=CARTESIAN_POINT('Origin',(3.,-7.5,108.25));
#43884=CARTESIAN_POINT('',(3.,-7.25665144929384,108.25));
#43885=CARTESIAN_POINT('',(3.,-7.5,107.845));
#43886=CARTESIAN_POINT('Origin',(-8.5,0.,109.576823573099));
#43887=CARTESIAN_POINT('',(-8.5,0.,109.453647146199));
#43888=CARTESIAN_POINT('',(-8.705,-2.51052593825207E-17,109.576823573099));
#43889=CARTESIAN_POINT('Origin',(7.,-8.65,127.));
#43890=CARTESIAN_POINT('',(6.5,-8.65,127.));
#43891=CARTESIAN_POINT('Origin',(6.3,-5.9,128.));
#43892=CARTESIAN_POINT('',(5.8,-5.9,128.));
#43893=CARTESIAN_POINT('',(6.3,-5.9,128.5));
#43894=CARTESIAN_POINT('Origin',(7.,-6.05,128.5));
#43895=CARTESIAN_POINT('',(7.7,-6.2,128.5));
#43896=CARTESIAN_POINT('Origin',(7.7,-6.2,128.));
#43897=CARTESIAN_POINT('',(8.2,-6.2,128.));
#43898=CARTESIAN_POINT('Origin',(7.,-6.05,123.5));
#43899=CARTESIAN_POINT('',(8.2,-6.06752483470939,123.5));
#43900=CARTESIAN_POINT('',(8.2,-6.35,123.5));
#43901=CARTESIAN_POINT('Origin',(7.,-7.2,123.5));
#43902=CARTESIAN_POINT('Origin',(8.2,-6.35,123.5));
#43903=CARTESIAN_POINT('',(8.2,-6.775,123.5));
#43904=CARTESIAN_POINT('Origin',(5.8,-5.75,123.5));
#43905=CARTESIAN_POINT('',(5.8,-6.475,123.5));
#43906=CARTESIAN_POINT('Origin',(7.,-7.2,123.5));
#43907=CARTESIAN_POINT('Origin',(7.,-7.2,123.5));
#43908=CARTESIAN_POINT('Origin',(7.,-8.35,123.5));
#43909=CARTESIAN_POINT('',(6.21259921259879,-8.65,123.5));
#43910=CARTESIAN_POINT('Origin',(7.,-7.2,123.5));
#43911=CARTESIAN_POINT('',(5.8,-8.65,123.5));
#43912=CARTESIAN_POINT('Origin',(5.8,-8.65,123.5));
#43913=CARTESIAN_POINT('',(6.4,-8.65,123.5));
#43914=CARTESIAN_POINT('Origin',(7.,-7.2,123.5));
#43915=CARTESIAN_POINT('Origin',(7.,-7.2,123.5));
#43916=CARTESIAN_POINT('Origin',(7.,-7.2,123.5));
#43917=CARTESIAN_POINT('',(5.35,-7.2,123.5));
#43918=CARTESIAN_POINT('Origin',(7.,-7.2,123.5));
#43919=CARTESIAN_POINT('Origin',(7.,-7.2,123.5));
#43920=CARTESIAN_POINT('Origin',(7.,-7.2,123.5));
#43921=CARTESIAN_POINT('Origin',(7.,-7.2,123.425));
#43922=CARTESIAN_POINT('',(5.2,-7.2,123.35));
#43923=CARTESIAN_POINT('',(5.275,-7.2,123.425));
#43924=CARTESIAN_POINT('Origin',(7.,-7.2,123.35));
#43925=CARTESIAN_POINT('Origin',(7.,-7.2,109.4));
#43926=CARTESIAN_POINT('',(5.2,-7.2,109.4));
#43927=CARTESIAN_POINT('Origin',(0.,0.,129.45));
#43928=CARTESIAN_POINT('',(-2.755,-3.37390193165096E-16,129.5));
#43929=CARTESIAN_POINT('Origin',(0.,0.,129.5));
#43930=CARTESIAN_POINT('',(-2.655,3.25143725173622E-16,129.4));
#43931=CARTESIAN_POINT('',(-2.705,-3.31266959169359E-16,129.45));
#43932=CARTESIAN_POINT('Origin',(0.,0.,129.4));
#43933=CARTESIAN_POINT('Origin',(0.,0.,120.275));
#43934=CARTESIAN_POINT('',(-2.655,-3.25143725173622E-16,111.));
#43935=CARTESIAN_POINT('Origin',(0.,0.,111.));
#43936=CARTESIAN_POINT('',(-2.655,-3.25143725173622E-16,120.275));
#43937=CARTESIAN_POINT('Origin',(0.,0.,129.5));
#43938=CARTESIAN_POINT('',(-5.29999999999999,-6.49062803548096E-16,129.5));
#43939=CARTESIAN_POINT('Origin',(0.,0.,129.5));
#43940=CARTESIAN_POINT('Origin',(4.85,0.,124.9));
#43941=CARTESIAN_POINT('Origin',(0.,0.,124.9));
#43942=CARTESIAN_POINT('Origin',(5.05,0.,124.5));
#43943=CARTESIAN_POINT('Origin',(0.,0.,124.5));
#43944=CARTESIAN_POINT('Origin',(2.655,0.,111.));
#43945=CARTESIAN_POINT('Origin',(0.,0.,109.9));
#43946=CARTESIAN_POINT('',(-5.,6.12323399573677E-16,109.9));
#43947=CARTESIAN_POINT('',(5.,-6.12323399573677E-16,109.9));
#43948=CARTESIAN_POINT('Origin',(0.,0.,109.9));
#43949=CARTESIAN_POINT('Origin',(5.4,-6.61309271539571E-16,109.9));
#43950=CARTESIAN_POINT('Origin',(0.,0.,109.9));
#43951=CARTESIAN_POINT('Origin',(0.,0.,118.45));
#43952=CARTESIAN_POINT('',(-5.,-6.12323399573677E-16,127.5));
#43953=CARTESIAN_POINT('Origin',(0.,0.,127.5));
#43954=CARTESIAN_POINT('',(-5.,-6.12323399573677E-16,118.45));
#43955=CARTESIAN_POINT('Origin',(5.3,0.,127.5));
#43956=CARTESIAN_POINT('',(-5.3,-6.49062803548097E-16,127.5));
#43957=CARTESIAN_POINT('Origin',(0.,0.,127.5));
#43958=CARTESIAN_POINT('Origin',(0.,0.,127.55));
#43959=CARTESIAN_POINT('',(-5.4,-6.61309271539571E-16,127.6));
#43960=CARTESIAN_POINT('Origin',(0.,0.,127.6));
#43961=CARTESIAN_POINT('',(-5.35,-6.55186037543834E-16,127.55));
#43962=CARTESIAN_POINT('Origin',(0.,0.,128.5));
#43963=CARTESIAN_POINT('',(-5.4,-6.61309271539571E-16,129.4));
#43964=CARTESIAN_POINT('Origin',(0.,0.,129.4));
#43965=CARTESIAN_POINT('',(-5.4,-6.61309271539571E-16,128.5));
#43966=CARTESIAN_POINT('Origin',(0.,0.,129.45));
#43967=CARTESIAN_POINT('',(-5.35,-6.55186037543834E-16,129.45));
#43968=CARTESIAN_POINT('Origin',(10.45,-5.375,107.05));
#43969=CARTESIAN_POINT('',(10.4,6.,107.));
#43970=CARTESIAN_POINT('',(10.4,6.,107.));
#43971=CARTESIAN_POINT('',(10.4,-8.5,107.));
#43972=CARTESIAN_POINT('',(10.5,-8.5,107.1));
#43973=CARTESIAN_POINT('',(10.4,-5.375,107.));
#43974=CARTESIAN_POINT('Origin',(9.5,6.,107.05));
#43975=CARTESIAN_POINT('',(9.5,6.9,107.));
#43976=CARTESIAN_POINT('',(9.5,6.9,107.));
#43977=CARTESIAN_POINT('Origin',(9.5,6.,107.));
#43978=CARTESIAN_POINT('Origin',(5.25,6.95,107.05));
#43979=CARTESIAN_POINT('',(-9.5,6.9,107.));
#43980=CARTESIAN_POINT('',(-9.5,7.,107.1));
#43981=CARTESIAN_POINT('',(-9.5,6.9,107.));
#43982=CARTESIAN_POINT('',(5.25,7.,107.1));
#43983=CARTESIAN_POINT('',(5.25,6.9,107.));
#43984=CARTESIAN_POINT('Origin',(-9.5,6.,107.05));
#43985=CARTESIAN_POINT('',(-10.4,6.,107.));
#43986=CARTESIAN_POINT('',(-10.5,6.,107.1));
#43987=CARTESIAN_POINT('',(-10.4,6.,107.));
#43988=CARTESIAN_POINT('Origin',(-9.5,6.,107.1));
#43989=CARTESIAN_POINT('Origin',(-9.5,6.,107.));
#43990=CARTESIAN_POINT('Origin',(-10.45,2.875,107.05));
#43991=CARTESIAN_POINT('',(-10.4,-8.5,107.));
#43992=CARTESIAN_POINT('',(-10.5,-8.5,107.1));
#43993=CARTESIAN_POINT('',(-10.4,-8.5,107.));
#43994=CARTESIAN_POINT('',(-10.5,2.875,107.1));
#43995=CARTESIAN_POINT('',(-10.4,2.875,107.));
#43996=CARTESIAN_POINT('Origin',(-9.5,-8.5,107.05));
#43997=CARTESIAN_POINT('',(-9.5,-9.4,107.));
#43998=CARTESIAN_POINT('',(-9.5,-9.4,107.));
#43999=CARTESIAN_POINT('Origin',(-9.5,-8.5,107.1));
#44000=CARTESIAN_POINT('Origin',(-9.5,-8.5,107.));
#44001=CARTESIAN_POINT('Origin',(-5.25,-9.45,107.05));
#44002=CARTESIAN_POINT('',(9.5,-9.4,107.));
#44003=CARTESIAN_POINT('',(9.5,-9.4,107.));
#44004=CARTESIAN_POINT('',(-5.25,-9.4,107.));
#44005=CARTESIAN_POINT('Origin',(9.5,-8.5,107.05));
#44006=CARTESIAN_POINT('Origin',(9.5,-8.5,107.));
#44007=CARTESIAN_POINT('Origin',(-9.5,-8.5,107.));
#44008=CARTESIAN_POINT('',(-10.5,-8.5,107.));
#44009=CARTESIAN_POINT('Origin',(0.,-1.25,107.));
#44010=CARTESIAN_POINT('Origin',(5.25,6.85,109.35));
#44011=CARTESIAN_POINT('',(9.5,6.7,109.5));
#44012=CARTESIAN_POINT('Origin',(9.5,6.,109.35));
#44013=CARTESIAN_POINT('Origin',(-10.5,7.,107.));
#44014=CARTESIAN_POINT('',(-10.5,6.,107.));
#44015=CARTESIAN_POINT('Origin',(-9.5,6.,107.));
#44016=CARTESIAN_POINT('',(-9.5,7.,107.));
#44017=CARTESIAN_POINT('Origin',(10.5,7.,107.));
#71456=UNCERTAINTY_MEASURE_WITH_UNIT(LENGTH_MEASURE(0.001),#71493,
'DISTANCE_ACCURACY_VALUE',
'Maximum model space distance between geometric entities at asserted c
onnectivities');
#71471=UNCERTAINTY_MEASURE_WITH_UNIT(LENGTH_MEASURE(0.001),#71493,
'DISTANCE_ACCURACY_VALUE',
'Maximum model space distance between geometric entities at asserted c
onnectivities');
#71477=(
GEOMETRIC_REPRESENTATION_CONTEXT(3)
GLOBAL_UNCERTAINTY_ASSIGNED_CONTEXT((#71456))
GLOBAL_UNIT_ASSIGNED_CONTEXT((#71493,#71495,#71496))
REPRESENTATION_CONTEXT('','3D')
);
#71492=(
GEOMETRIC_REPRESENTATION_CONTEXT(3)
GLOBAL_UNCERTAINTY_ASSIGNED_CONTEXT((#71471))
GLOBAL_UNIT_ASSIGNED_CONTEXT((#71493,#71495,#71496))
REPRESENTATION_CONTEXT('','3D')
);
#71493=(
LENGTH_UNIT()
NAMED_UNIT(*)
SI_UNIT(.CENTI.,.METRE.)
);
#71495=(
NAMED_UNIT(*)
PLANE_ANGLE_UNIT()
SI_UNIT($,.RADIAN.)
);
#71496=(
NAMED_UNIT(*)
SI_UNIT($,.STERADIAN.)
SOLID_ANGLE_UNIT()
);
#71502=SHAPE_DEFINITION_REPRESENTATION(#71522,#71607);
#71522=PRODUCT_DEFINITION_SHAPE('',$,#71628);
#71607=SHAPE_REPRESENTATION('',(#29346),#71477);
#71622=PRODUCT_DEFINITION_CONTEXT('part definition',#71684,'design');
#71628=PRODUCT_DEFINITION('2026-10-19-03-22-09-909',
'09_Bottle_Jack_Body_20T_Hand_Pump',#71648,#71622);
#71648=PRODUCT_DEFINITION_FORMATION('',$,#71691);
#71684=APPLICATION_CONTEXT(
'Core Data for Automotive Mechanical Design Process');
#71685=PRODUCT_CONTEXT('part definition',#71684,'mechanical');
#71691=PRODUCT('2026-10-19-03-22-09-909',
'09_Bottle_Jack_Body_20T_Hand_Pump',$,(#71685));
#71860=COLOUR_RGB('Dark Blue',0.08,0.2,0.34);
#71861=FILL_AREA_STYLE_COLOUR('',#71860);
#71862=FILL_AREA_STYLE('',(#71861));
#71863=SURFACE_STYLE_FILL_AREA(#71862);
#71864=SURFACE_SIDE_STYLE('',(#71863));
#71865=SURFACE_STYLE_USAGE(.BOTH.,#71864);
#71866=PRESENTATION_STYLE_ASSIGNMENT((#71865));
ENDSEC;
END-ISO-10303-21;
